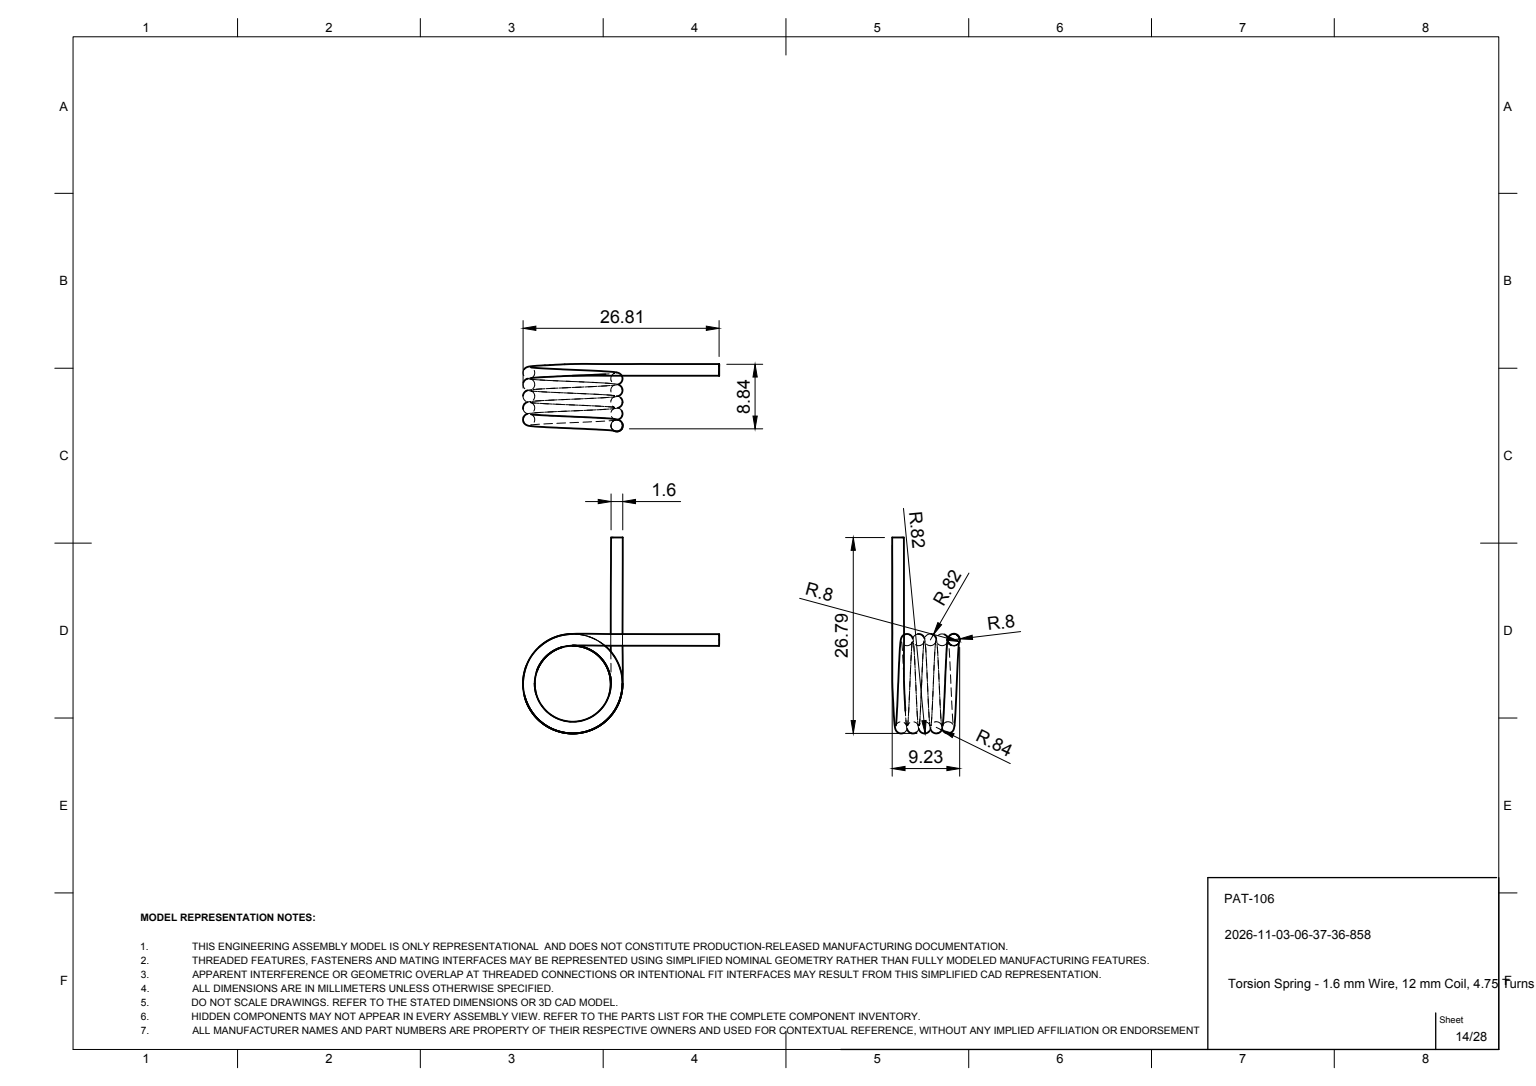
ISO-10303-21;
HEADER;
/* Generated by software containing ST-Developer
 * from STEP Tools, Inc. (www.steptools.com) 
 */

FILE_DESCRIPTION(
/* description */ ('Torsion-spring ratchet demonstrator'),
/* implementation_level */ '2;1');

FILE_NAME(
/* name */ 'Torsion Spring - 1.6 mm Wire, 12 mm Coil, 4.75 Turns.step',
/* time_stamp */ '2026-10-29T17:29:17-07:00',
/* author */ (''),
/* organization */ (''),
/* preprocessor_version */ 'ST-DEVELOPER v20.2',
/* originating_system */ 'Autodesk Translation Framework v15.17.0.0',
/* authorisation */ '');

FILE_SCHEMA (('AUTOMOTIVE_DESIGN { 1 0 10303 214 3 1 1 }'));
ENDSEC;

DATA;
#10=MECHANICAL_DESIGN_GEOMETRIC_PRESENTATION_REPRESENTATION('',(#307),#11258);
#11=B_SPLINE_SURFACE_WITH_KNOTS('',3,3,((#8927,#8928,#8929,#8930,#8931,
#8932,#8933,#8934,#8935,#8936,#8937,#8938,#8939,#8940,#8941,#8942,#8943,
#8944,#8945,#8946,#8947,#8948,#8949,#8950,#8951,#8952,#8953,#8954,#8955,
#8956,#8957,#8958,#8959,#8960,#8961,#8962,#8963,#8964,#8965,#8966,#8967,
#8968,#8969,#8970,#8971,#8972,#8973,#8974,#8975,#8976,#8977,#8978,#8979,
#8980,#8981,#8982,#8983,#8984,#8985,#8986,#8987,#8988,#8989,#8990,#8991,
#8992,#8993),(#8994,#8995,#8996,#8997,#8998,#8999,#9000,#9001,#9002,#9003,
#9004,#9005,#9006,#9007,#9008,#9009,#9010,#9011,#9012,#9013,#9014,#9015,
#9016,#9017,#9018,#9019,#9020,#9021,#9022,#9023,#9024,#9025,#9026,#9027,
#9028,#9029,#9030,#9031,#9032,#9033,#9034,#9035,#9036,#9037,#9038,#9039,
#9040,#9041,#9042,#9043,#9044,#9045,#9046,#9047,#9048,#9049,#9050,#9051,
#9052,#9053,#9054,#9055,#9056,#9057,#9058,#9059,#9060),(#9061,#9062,#9063,
#9064,#9065,#9066,#9067,#9068,#9069,#9070,#9071,#9072,#9073,#9074,#9075,
#9076,#9077,#9078,#9079,#9080,#9081,#9082,#9083,#9084,#9085,#9086,#9087,
#9088,#9089,#9090,#9091,#9092,#9093,#9094,#9095,#9096,#9097,#9098,#9099,
#9100,#9101,#9102,#9103,#9104,#9105,#9106,#9107,#9108,#9109,#9110,#9111,
#9112,#9113,#9114,#9115,#9116,#9117,#9118,#9119,#9120,#9121,#9122,#9123,
#9124,#9125,#9126,#9127),(#9128,#9129,#9130,#9131,#9132,#9133,#9134,#9135,
#9136,#9137,#9138,#9139,#9140,#9141,#9142,#9143,#9144,#9145,#9146,#9147,
#9148,#9149,#9150,#9151,#9152,#9153,#9154,#9155,#9156,#9157,#9158,#9159,
#9160,#9161,#9162,#9163,#9164,#9165,#9166,#9167,#9168,#9169,#9170,#9171,
#9172,#9173,#9174,#9175,#9176,#9177,#9178,#9179,#9180,#9181,#9182,#9183,
#9184,#9185,#9186,#9187,#9188,#9189,#9190,#9191,#9192,#9193,#9194),(#9195,
#9196,#9197,#9198,#9199,#9200,#9201,#9202,#9203,#9204,#9205,#9206,#9207,
#9208,#9209,#9210,#9211,#9212,#9213,#9214,#9215,#9216,#9217,#9218,#9219,
#9220,#9221,#9222,#9223,#9224,#9225,#9226,#9227,#9228,#9229,#9230,#9231,
#9232,#9233,#9234,#9235,#9236,#9237,#9238,#9239,#9240,#9241,#9242,#9243,
#9244,#9245,#9246,#9247,#9248,#9249,#9250,#9251,#9252,#9253,#9254,#9255,
#9256,#9257,#9258,#9259,#9260,#9261),(#9262,#9263,#9264,#9265,#9266,#9267,
#9268,#9269,#9270,#9271,#9272,#9273,#9274,#9275,#9276,#9277,#9278,#9279,
#9280,#9281,#9282,#9283,#9284,#9285,#9286,#9287,#9288,#9289,#9290,#9291,
#9292,#9293,#9294,#9295,#9296,#9297,#9298,#9299,#9300,#9301,#9302,#9303,
#9304,#9305,#9306,#9307,#9308,#9309,#9310,#9311,#9312,#9313,#9314,#9315,
#9316,#9317,#9318,#9319,#9320,#9321,#9322,#9323,#9324,#9325,#9326,#9327,
#9328),(#9329,#9330,#9331,#9332,#9333,#9334,#9335,#9336,#9337,#9338,#9339,
#9340,#9341,#9342,#9343,#9344,#9345,#9346,#9347,#9348,#9349,#9350,#9351,
#9352,#9353,#9354,#9355,#9356,#9357,#9358,#9359,#9360,#9361,#9362,#9363,
#9364,#9365,#9366,#9367,#9368,#9369,#9370,#9371,#9372,#9373,#9374,#9375,
#9376,#9377,#9378,#9379,#9380,#9381,#9382,#9383,#9384,#9385,#9386,#9387,
#9388,#9389,#9390,#9391,#9392,#9393,#9394,#9395),(#9396,#9397,#9398,#9399,
#9400,#9401,#9402,#9403,#9404,#9405,#9406,#9407,#9408,#9409,#9410,#9411,
#9412,#9413,#9414,#9415,#9416,#9417,#9418,#9419,#9420,#9421,#9422,#9423,
#9424,#9425,#9426,#9427,#9428,#9429,#9430,#9431,#9432,#9433,#9434,#9435,
#9436,#9437,#9438,#9439,#9440,#9441,#9442,#9443,#9444,#9445,#9446,#9447,
#9448,#9449,#9450,#9451,#9452,#9453,#9454,#9455,#9456,#9457,#9458,#9459,
#9460,#9461,#9462),(#9463,#9464,#9465,#9466,#9467,#9468,#9469,#9470,#9471,
#9472,#9473,#9474,#9475,#9476,#9477,#9478,#9479,#9480,#9481,#9482,#9483,
#9484,#9485,#9486,#9487,#9488,#9489,#9490,#9491,#9492,#9493,#9494,#9495,
#9496,#9497,#9498,#9499,#9500,#9501,#9502,#9503,#9504,#9505,#9506,#9507,
#9508,#9509,#9510,#9511,#9512,#9513,#9514,#9515,#9516,#9517,#9518,#9519,
#9520,#9521,#9522,#9523,#9524,#9525,#9526,#9527,#9528,#9529)),
 .UNSPECIFIED.,.F.,.F.,.F.,(4,1,1,1,1,1,4),(4,1,1,1,1,1,1,1,1,1,1,1,1,1,
1,1,1,1,1,1,1,1,1,1,1,1,1,1,1,1,1,1,1,1,1,1,1,1,1,1,1,1,1,1,1,1,1,1,1,1,
1,1,1,1,1,1,1,1,1,1,1,1,1,1,4),(-2.2472005777546,-1.52802098913967,-0.808841400524738,
-0.329388341448117,0.150064717628504,0.629517776705124,1.10897083578174),
(0.,0.0178571428571429,0.0357142857142857,0.0446428571428571,0.0535714285714286,
0.0625,0.0714285714285714,0.0803571428571428,0.0848214285714286,0.0892857142857143,
0.0982142857142857,0.107142857142857,0.125,0.142857142857143,0.166666666666667,
0.19047619047619,0.214285714285714,0.232142857142857,0.25,0.267857142857143,
0.285714285714286,0.303571428571429,0.321428571428571,0.339285714285714,
0.357142857142857,0.369047619047619,0.392857142857143,0.410714285714286,
0.428571428571429,0.452380952380952,0.476190476190476,0.492063492063492,
0.507936507936508,0.523809523809524,0.547619047619048,0.571428571428571,
0.595238095238095,0.619047619047619,0.642857142857143,0.666666666666667,
0.682539682539682,0.698412698412698,0.714285714285714,0.73015873015873,
0.746031746031746,0.761904761904762,0.785714285714286,0.809523809523809,
0.833333333333333,0.857142857142857,0.861607142857143,0.866071428571429,
0.875,0.892857142857143,0.901785714285714,0.910714285714286,0.915178571428571,
0.919642857142857,0.928571428571429,0.9375,0.946428571428571,0.955357142857143,
0.964285714285714,0.982142857142857,1.),.UNSPECIFIED.);
#12=B_SPLINE_SURFACE_WITH_KNOTS('',3,3,((#9670,#9671,#9672,#9673,#9674,
#9675,#9676,#9677,#9678,#9679,#9680,#9681,#9682,#9683,#9684,#9685,#9686,
#9687,#9688,#9689,#9690,#9691,#9692,#9693,#9694,#9695,#9696,#9697,#9698,
#9699,#9700,#9701,#9702,#9703,#9704,#9705,#9706,#9707,#9708,#9709,#9710,
#9711,#9712,#9713,#9714,#9715,#9716,#9717,#9718,#9719,#9720,#9721,#9722,
#9723,#9724,#9725,#9726,#9727,#9728,#9729,#9730,#9731,#9732,#9733,#9734,
#9735,#9736,#9737,#9738,#9739,#9740),(#9741,#9742,#9743,#9744,#9745,#9746,
#9747,#9748,#9749,#9750,#9751,#9752,#9753,#9754,#9755,#9756,#9757,#9758,
#9759,#9760,#9761,#9762,#9763,#9764,#9765,#9766,#9767,#9768,#9769,#9770,
#9771,#9772,#9773,#9774,#9775,#9776,#9777,#9778,#9779,#9780,#9781,#9782,
#9783,#9784,#9785,#9786,#9787,#9788,#9789,#9790,#9791,#9792,#9793,#9794,
#9795,#9796,#9797,#9798,#9799,#9800,#9801,#9802,#9803,#9804,#9805,#9806,
#9807,#9808,#9809,#9810,#9811),(#9812,#9813,#9814,#9815,#9816,#9817,#9818,
#9819,#9820,#9821,#9822,#9823,#9824,#9825,#9826,#9827,#9828,#9829,#9830,
#9831,#9832,#9833,#9834,#9835,#9836,#9837,#9838,#9839,#9840,#9841,#9842,
#9843,#9844,#9845,#9846,#9847,#9848,#9849,#9850,#9851,#9852,#9853,#9854,
#9855,#9856,#9857,#9858,#9859,#9860,#9861,#9862,#9863,#9864,#9865,#9866,
#9867,#9868,#9869,#9870,#9871,#9872,#9873,#9874,#9875,#9876,#9877,#9878,
#9879,#9880,#9881,#9882),(#9883,#9884,#9885,#9886,#9887,#9888,#9889,#9890,
#9891,#9892,#9893,#9894,#9895,#9896,#9897,#9898,#9899,#9900,#9901,#9902,
#9903,#9904,#9905,#9906,#9907,#9908,#9909,#9910,#9911,#9912,#9913,#9914,
#9915,#9916,#9917,#9918,#9919,#9920,#9921,#9922,#9923,#9924,#9925,#9926,
#9927,#9928,#9929,#9930,#9931,#9932,#9933,#9934,#9935,#9936,#9937,#9938,
#9939,#9940,#9941,#9942,#9943,#9944,#9945,#9946,#9947,#9948,#9949,#9950,
#9951,#9952,#9953)),.UNSPECIFIED.,.F.,.F.,.F.,(4,4),(4,1,1,1,1,1,1,1,1,
1,1,1,1,1,1,1,1,1,1,1,1,1,1,1,1,1,1,1,1,1,1,1,1,1,1,1,1,1,1,1,1,1,1,1,1,
1,1,1,1,1,1,1,1,1,1,1,1,1,1,1,1,1,1,1,1,1,1,1,4),(3.14159265358979,4.03598472942499),
(0.,0.0178571428571429,0.0357142857142857,0.0446428571428571,0.0535714285714286,
0.0625,0.0714285714285714,0.0803571428571428,0.0892857142857143,0.0982142857142857,
0.107142857142857,0.125,0.142857142857143,0.166666666666667,0.19047619047619,
0.196428571428571,0.214285714285714,0.232142857142857,0.25,0.267857142857143,
0.285714285714286,0.303571428571429,0.321428571428571,0.339285714285714,
0.357142857142857,0.369047619047619,0.392857142857143,0.410714285714286,
0.419642857142857,0.428571428571429,0.452380952380952,0.476190476190476,
0.492063492063492,0.5,0.507936507936508,0.523809523809524,0.547619047619048,
0.571428571428571,0.595238095238095,0.619047619047619,0.642857142857143,
0.666666666666667,0.682539682539682,0.698412698412698,0.714285714285714,
0.722222222222222,0.73015873015873,0.746031746031746,0.761904761904762,
0.773809523809524,0.785714285714286,0.809523809523809,0.833333333333333,
0.857142857142857,0.859375,0.861607142857143,0.866071428571429,0.875,0.892857142857143,
0.901785714285714,0.910714285714286,0.919642857142857,0.928571428571429,
0.9375,0.946428571428571,0.955357142857143,0.964285714285714,0.982142857142857,
1.),.UNSPECIFIED.);
#13=B_SPLINE_SURFACE_WITH_KNOTS('',3,3,((#10029,#10030,#10031,#10032,#10033,
#10034,#10035,#10036,#10037,#10038,#10039,#10040,#10041,#10042,#10043,#10044,
#10045,#10046,#10047,#10048,#10049,#10050,#10051,#10052,#10053,#10054,#10055,
#10056,#10057,#10058,#10059,#10060,#10061,#10062,#10063,#10064,#10065,#10066,
#10067,#10068,#10069,#10070,#10071,#10072,#10073,#10074,#10075,#10076,#10077,
#10078,#10079,#10080,#10081,#10082,#10083,#10084,#10085,#10086,#10087,#10088,
#10089,#10090,#10091,#10092,#10093,#10094,#10095,#10096,#10097,#10098,#10099,
#10100),(#10101,#10102,#10103,#10104,#10105,#10106,#10107,#10108,#10109,
#10110,#10111,#10112,#10113,#10114,#10115,#10116,#10117,#10118,#10119,#10120,
#10121,#10122,#10123,#10124,#10125,#10126,#10127,#10128,#10129,#10130,#10131,
#10132,#10133,#10134,#10135,#10136,#10137,#10138,#10139,#10140,#10141,#10142,
#10143,#10144,#10145,#10146,#10147,#10148,#10149,#10150,#10151,#10152,#10153,
#10154,#10155,#10156,#10157,#10158,#10159,#10160,#10161,#10162,#10163,#10164,
#10165,#10166,#10167,#10168,#10169,#10170,#10171,#10172),(#10173,#10174,
#10175,#10176,#10177,#10178,#10179,#10180,#10181,#10182,#10183,#10184,#10185,
#10186,#10187,#10188,#10189,#10190,#10191,#10192,#10193,#10194,#10195,#10196,
#10197,#10198,#10199,#10200,#10201,#10202,#10203,#10204,#10205,#10206,#10207,
#10208,#10209,#10210,#10211,#10212,#10213,#10214,#10215,#10216,#10217,#10218,
#10219,#10220,#10221,#10222,#10223,#10224,#10225,#10226,#10227,#10228,#10229,
#10230,#10231,#10232,#10233,#10234,#10235,#10236,#10237,#10238,#10239,#10240,
#10241,#10242,#10243,#10244),(#10245,#10246,#10247,#10248,#10249,#10250,
#10251,#10252,#10253,#10254,#10255,#10256,#10257,#10258,#10259,#10260,#10261,
#10262,#10263,#10264,#10265,#10266,#10267,#10268,#10269,#10270,#10271,#10272,
#10273,#10274,#10275,#10276,#10277,#10278,#10279,#10280,#10281,#10282,#10283,
#10284,#10285,#10286,#10287,#10288,#10289,#10290,#10291,#10292,#10293,#10294,
#10295,#10296,#10297,#10298,#10299,#10300,#10301,#10302,#10303,#10304,#10305,
#10306,#10307,#10308,#10309,#10310,#10311,#10312,#10313,#10314,#10315,#10316),
(#10317,#10318,#10319,#10320,#10321,#10322,#10323,#10324,#10325,#10326,
#10327,#10328,#10329,#10330,#10331,#10332,#10333,#10334,#10335,#10336,#10337,
#10338,#10339,#10340,#10341,#10342,#10343,#10344,#10345,#10346,#10347,#10348,
#10349,#10350,#10351,#10352,#10353,#10354,#10355,#10356,#10357,#10358,#10359,
#10360,#10361,#10362,#10363,#10364,#10365,#10366,#10367,#10368,#10369,#10370,
#10371,#10372,#10373,#10374,#10375,#10376,#10377,#10378,#10379,#10380,#10381,
#10382,#10383,#10384,#10385,#10386,#10387,#10388),(#10389,#10390,#10391,
#10392,#10393,#10394,#10395,#10396,#10397,#10398,#10399,#10400,#10401,#10402,
#10403,#10404,#10405,#10406,#10407,#10408,#10409,#10410,#10411,#10412,#10413,
#10414,#10415,#10416,#10417,#10418,#10419,#10420,#10421,#10422,#10423,#10424,
#10425,#10426,#10427,#10428,#10429,#10430,#10431,#10432,#10433,#10434,#10435,
#10436,#10437,#10438,#10439,#10440,#10441,#10442,#10443,#10444,#10445,#10446,
#10447,#10448,#10449,#10450,#10451,#10452,#10453,#10454,#10455,#10456,#10457,
#10458,#10459,#10460)),.UNSPECIFIED.,.F.,.F.,.F.,(4,1,1,4),(4,1,1,1,1,1,
1,1,1,1,1,1,1,1,1,1,1,1,1,1,1,1,1,1,1,1,1,1,1,1,1,1,1,1,1,1,1,1,1,1,1,1,
1,1,1,1,1,1,1,1,1,1,1,1,1,1,1,1,1,1,1,1,1,1,1,1,1,1,1,4),(1.10897083578174,
1.98009447198525,2.56084356278759,3.14159265358993),(0.,0.0178571428571429,
0.0357142857142857,0.0446428571428571,0.0535714285714286,0.0625,0.0714285714285714,
0.0803571428571428,0.0848214285714286,0.0892857142857143,0.0982142857142857,
0.107142857142857,0.125,0.142857142857143,0.166666666666667,0.19047619047619,
0.196428571428571,0.214285714285714,0.232142857142857,0.25,0.267857142857143,
0.285714285714286,0.303571428571429,0.321428571428571,0.339285714285714,
0.357142857142857,0.369047619047619,0.392857142857143,0.410714285714286,
0.419642857142857,0.428571428571429,0.452380952380952,0.476190476190476,
0.492063492063492,0.507936507936508,0.523809523809524,0.547619047619048,
0.571428571428571,0.595238095238095,0.619047619047619,0.642857142857143,
0.666666666666667,0.682539682539682,0.698412698412698,0.714285714285714,
0.73015873015873,0.746031746031746,0.761904761904762,0.773809523809524,
0.785714285714286,0.791666666666667,0.809523809523809,0.833333333333333,
0.857142857142857,0.859375,0.861607142857143,0.866071428571429,0.875,0.892857142857143,
0.901785714285714,0.910714285714286,0.915178571428571,0.919642857142857,
0.928571428571429,0.9375,0.946428571428571,0.955357142857143,0.964285714285714,
0.982142857142857,1.),.UNSPECIFIED.);
#223=B_SPLINE_CURVE_WITH_KNOTS('',3,(#9532,#9533,#9534,#9535,#9536,#9537,
#9538,#9539,#9540,#9541,#9542,#9543,#9544,#9545,#9546,#9547,#9548,#9549,
#9550,#9551,#9552,#9553,#9554,#9555,#9556,#9557,#9558,#9559,#9560,#9561,
#9562,#9563,#9564,#9565,#9566,#9567,#9568,#9569,#9570,#9571,#9572,#9573,
#9574,#9575,#9576,#9577,#9578,#9579,#9580,#9581,#9582,#9583,#9584,#9585,
#9586,#9587,#9588,#9589,#9590,#9591,#9592,#9593,#9594,#9595,#9596,#9597,
#9598),.UNSPECIFIED.,.F.,.F.,(4,1,1,1,1,1,1,1,1,1,1,1,1,1,1,1,1,1,1,1,1,
1,1,1,1,1,1,1,1,1,1,1,1,1,1,1,1,1,1,1,1,1,1,1,1,1,1,1,1,1,1,1,1,1,1,1,1,
1,1,1,1,1,1,1,4),(-1.,-0.982142857142857,-0.964285714285714,-0.955357142857143,
-0.946428571428571,-0.9375,-0.928571428571429,-0.919642857142857,-0.915178571428571,
-0.910714285714286,-0.901785714285714,-0.892857142857143,-0.875,-0.866071428571429,
-0.861607142857143,-0.857142857142857,-0.833333333333333,-0.809523809523809,
-0.785714285714286,-0.761904761904762,-0.746031746031746,-0.73015873015873,
-0.714285714285714,-0.698412698412698,-0.682539682539682,-0.666666666666667,
-0.642857142857143,-0.619047619047619,-0.595238095238095,-0.571428571428571,
-0.547619047619048,-0.523809523809524,-0.507936507936508,-0.492063492063492,
-0.476190476190476,-0.452380952380952,-0.428571428571429,-0.410714285714286,
-0.392857142857143,-0.369047619047619,-0.357142857142857,-0.339285714285714,
-0.321428571428571,-0.303571428571429,-0.285714285714286,-0.267857142857143,
-0.25,-0.232142857142857,-0.214285714285714,-0.19047619047619,-0.166666666666667,
-0.142857142857143,-0.125,-0.107142857142857,-0.0982142857142857,-0.0892857142857143,
-0.0848214285714286,-0.0803571428571428,-0.0714285714285714,-0.0625,-0.0535714285714286,
-0.0446428571428571,-0.0357142857142857,-0.0178571428571429,0.),
 .UNSPECIFIED.);
#224=B_SPLINE_CURVE_WITH_KNOTS('',3,(#9602,#9603,#9604,#9605,#9606,#9607,
#9608,#9609,#9610,#9611,#9612,#9613,#9614,#9615,#9616,#9617,#9618,#9619,
#9620,#9621,#9622,#9623,#9624,#9625,#9626,#9627,#9628,#9629,#9630,#9631,
#9632,#9633,#9634,#9635,#9636,#9637,#9638,#9639,#9640,#9641,#9642,#9643,
#9644,#9645,#9646,#9647,#9648,#9649,#9650,#9651,#9652,#9653,#9654,#9655,
#9656,#9657,#9658,#9659,#9660,#9661,#9662,#9663,#9664,#9665,#9666,#9667,
#9668),.UNSPECIFIED.,.F.,.F.,(4,1,1,1,1,1,1,1,1,1,1,1,1,1,1,1,1,1,1,1,1,
1,1,1,1,1,1,1,1,1,1,1,1,1,1,1,1,1,1,1,1,1,1,1,1,1,1,1,1,1,1,1,1,1,1,1,1,
1,1,1,1,1,1,1,4),(-1.,-0.982142857142857,-0.964285714285714,-0.955357142857143,
-0.946428571428571,-0.9375,-0.928571428571429,-0.919642857142857,-0.915178571428571,
-0.910714285714286,-0.901785714285714,-0.892857142857143,-0.875,-0.866071428571429,
-0.861607142857143,-0.857142857142857,-0.833333333333333,-0.809523809523809,
-0.785714285714286,-0.761904761904762,-0.746031746031746,-0.73015873015873,
-0.714285714285714,-0.698412698412698,-0.682539682539682,-0.666666666666667,
-0.642857142857143,-0.619047619047619,-0.595238095238095,-0.571428571428571,
-0.547619047619048,-0.523809523809524,-0.507936507936508,-0.492063492063492,
-0.476190476190476,-0.452380952380952,-0.428571428571429,-0.410714285714286,
-0.392857142857143,-0.369047619047619,-0.357142857142857,-0.339285714285714,
-0.321428571428571,-0.303571428571429,-0.285714285714286,-0.267857142857143,
-0.25,-0.232142857142857,-0.214285714285714,-0.19047619047619,-0.166666666666667,
-0.142857142857143,-0.125,-0.107142857142857,-0.0982142857142857,-0.0892857142857143,
-0.0848214285714286,-0.0803571428571428,-0.0714285714285714,-0.0625,-0.0535714285714286,
-0.0446428571428571,-0.0357142857142857,-0.0178571428571429,0.),
 .UNSPECIFIED.);
#225=B_SPLINE_CURVE_WITH_KNOTS('',3,(#9957,#9958,#9959,#9960,#9961,#9962,
#9963,#9964,#9965,#9966,#9967,#9968,#9969,#9970,#9971,#9972,#9973,#9974,
#9975,#9976,#9977,#9978,#9979,#9980,#9981,#9982,#9983,#9984,#9985,#9986,
#9987,#9988,#9989,#9990,#9991,#9992,#9993,#9994,#9995,#9996,#9997,#9998,
#9999,#10000,#10001,#10002,#10003,#10004,#10005,#10006,#10007,#10008,#10009,
#10010,#10011,#10012,#10013,#10014,#10015,#10016,#10017,#10018,#10019,#10020,
#10021,#10022,#10023,#10024,#10025,#10026,#10027),.UNSPECIFIED.,.F.,.F.,
(4,1,1,1,1,1,1,1,1,1,1,1,1,1,1,1,1,1,1,1,1,1,1,1,1,1,1,1,1,1,1,1,1,1,1,
1,1,1,1,1,1,1,1,1,1,1,1,1,1,1,1,1,1,1,1,1,1,1,1,1,1,1,1,1,1,1,1,1,4),(0.,
0.0178571428571429,0.0357142857142857,0.0446428571428571,0.0535714285714286,
0.0625,0.0714285714285714,0.0803571428571428,0.0892857142857143,0.0982142857142857,
0.107142857142857,0.125,0.142857142857143,0.166666666666667,0.19047619047619,
0.196428571428571,0.214285714285714,0.232142857142857,0.25,0.267857142857143,
0.285714285714286,0.303571428571429,0.321428571428571,0.339285714285714,
0.357142857142857,0.369047619047619,0.392857142857143,0.410714285714286,
0.419642857142857,0.428571428571429,0.452380952380952,0.476190476190476,
0.492063492063492,0.5,0.507936507936508,0.523809523809524,0.547619047619048,
0.571428571428571,0.595238095238095,0.619047619047619,0.642857142857143,
0.666666666666667,0.682539682539682,0.698412698412698,0.714285714285714,
0.722222222222222,0.73015873015873,0.746031746031746,0.761904761904762,
0.773809523809524,0.785714285714286,0.809523809523809,0.833333333333333,
0.857142857142857,0.859375,0.861607142857143,0.866071428571429,0.875,0.892857142857143,
0.901785714285714,0.910714285714286,0.919642857142857,0.928571428571429,
0.9375,0.946428571428571,0.955357142857143,0.964285714285714,0.982142857142857,
1.),.UNSPECIFIED.);
#251=SHAPE_REPRESENTATION_RELATIONSHIP('SRR','None',#11378,#275);
#275=ADVANCED_BREP_SHAPE_REPRESENTATION('',(#337),#11248);
#307=STYLED_ITEM('',(#11584),#337);
#337=MANIFOLD_SOLID_BREP('Body1',#5180);
#528=PLANE('',#5869);
#529=PLANE('',#5870);
#810=FACE_OUTER_BOUND('',#1190,.T.);
#811=FACE_OUTER_BOUND('',#1191,.T.);
#812=FACE_OUTER_BOUND('',#1192,.T.);
#813=FACE_OUTER_BOUND('',#1193,.T.);
#814=FACE_OUTER_BOUND('',#1194,.T.);
#1190=EDGE_LOOP('',(#4194,#4195,#4196,#4197));
#1191=EDGE_LOOP('',(#4198,#4199,#4200,#4201));
#1192=EDGE_LOOP('',(#4202,#4203,#4204,#4205));
#1193=EDGE_LOOP('',(#4206,#4207,#4208));
#1194=EDGE_LOOP('',(#4209,#4210,#4211));
#2289=CIRCLE('',#5863,0.08);
#2290=CIRCLE('',#5864,0.08);
#2291=CIRCLE('',#5865,0.08);
#2292=CIRCLE('',#5866,0.08);
#2293=CIRCLE('',#5867,0.08);
#2294=CIRCLE('',#5868,0.08);
#2593=VERTEX_POINT('',#9530);
#2594=VERTEX_POINT('',#9531);
#2595=VERTEX_POINT('',#9599);
#2596=VERTEX_POINT('',#9601);
#2597=VERTEX_POINT('',#9954);
#2598=VERTEX_POINT('',#9956);
#3157=EDGE_CURVE('',#2593,#2594,#223,.T.);
#3158=EDGE_CURVE('',#2595,#2593,#2289,.T.);
#3159=EDGE_CURVE('',#2595,#2596,#224,.T.);
#3160=EDGE_CURVE('',#2596,#2594,#2290,.T.);
#3161=EDGE_CURVE('',#2597,#2595,#2291,.T.);
#3162=EDGE_CURVE('',#2598,#2597,#225,.T.);
#3163=EDGE_CURVE('',#2598,#2596,#2292,.T.);
#3164=EDGE_CURVE('',#2594,#2598,#2293,.T.);
#3165=EDGE_CURVE('',#2593,#2597,#2294,.T.);
#4194=ORIENTED_EDGE('',*,*,#3157,.F.);
#4195=ORIENTED_EDGE('',*,*,#3158,.F.);
#4196=ORIENTED_EDGE('',*,*,#3159,.T.);
#4197=ORIENTED_EDGE('',*,*,#3160,.T.);
#4198=ORIENTED_EDGE('',*,*,#3159,.F.);
#4199=ORIENTED_EDGE('',*,*,#3161,.F.);
#4200=ORIENTED_EDGE('',*,*,#3162,.F.);
#4201=ORIENTED_EDGE('',*,*,#3163,.T.);
#4202=ORIENTED_EDGE('',*,*,#3157,.T.);
#4203=ORIENTED_EDGE('',*,*,#3164,.T.);
#4204=ORIENTED_EDGE('',*,*,#3162,.T.);
#4205=ORIENTED_EDGE('',*,*,#3165,.F.);
#4206=ORIENTED_EDGE('',*,*,#3161,.T.);
#4207=ORIENTED_EDGE('',*,*,#3158,.T.);
#4208=ORIENTED_EDGE('',*,*,#3165,.T.);
#4209=ORIENTED_EDGE('',*,*,#3163,.F.);
#4210=ORIENTED_EDGE('',*,*,#3164,.F.);
#4211=ORIENTED_EDGE('',*,*,#3160,.F.);
#5036=ADVANCED_FACE('',(#810),#11,.T.);
#5037=ADVANCED_FACE('',(#811),#12,.T.);
#5038=ADVANCED_FACE('',(#812),#13,.T.);
#5039=ADVANCED_FACE('',(#813),#528,.T.);
#5040=ADVANCED_FACE('',(#814),#529,.F.);
#5180=CLOSED_SHELL('',(#5036,#5037,#5038,#5039,#5040));
#5862=AXIS2_PLACEMENT_3D('',#8926,#7040,#7041);
#5863=AXIS2_PLACEMENT_3D('',#9600,#7042,#7043);
#5864=AXIS2_PLACEMENT_3D('',#9669,#7044,#7045);
#5865=AXIS2_PLACEMENT_3D('',#9955,#7046,#7047);
#5866=AXIS2_PLACEMENT_3D('',#10028,#7048,#7049);
#5867=AXIS2_PLACEMENT_3D('',#10461,#7050,#7051);
#5868=AXIS2_PLACEMENT_3D('',#10462,#7052,#7053);
#5869=AXIS2_PLACEMENT_3D('',#10463,#7054,#7055);
#5870=AXIS2_PLACEMENT_3D('',#10464,#7056,#7057);
#7040=DIRECTION('axis',(0.,0.,1.));
#7041=DIRECTION('refdir',(1.,0.,0.));
#7042=DIRECTION('center_axis',(0.999998225160355,-0.00106218492982768,0.00155609746344814));
#7043=DIRECTION('ref_axis',(-0.00116547091797426,0.300191357997798,0.953878289018561));
#7044=DIRECTION('center_axis',(0.00155609740738298,-0.0010621849112801,
0.999998225160462));
#7045=DIRECTION('ref_axis',(-0.00155444353908754,0.999998225160461,0.0010646037811343));
#7046=DIRECTION('center_axis',(0.999998225160355,-0.00106218492982768,0.00155609746344814));
#7047=DIRECTION('ref_axis',(-0.00116547091797426,0.300191357997798,0.953878289018561));
#7048=DIRECTION('center_axis',(0.00155609740738298,-0.0010621849112801,
0.999998225160462));
#7049=DIRECTION('ref_axis',(-0.00155444353908754,0.999998225160461,0.0010646037811343));
#7050=DIRECTION('center_axis',(0.00155609740738298,-0.0010621849112801,
0.999998225160462));
#7051=DIRECTION('ref_axis',(-0.00155444353908754,0.999998225160461,0.0010646037811343));
#7052=DIRECTION('center_axis',(0.999998225160355,-0.00106218492982768,0.00155609746344814));
#7053=DIRECTION('ref_axis',(-0.00116547091797426,0.300191357997798,0.953878289018561));
#7054=DIRECTION('center_axis',(0.999998225160355,-0.00106218492982768,0.00155609746344814));
#7055=DIRECTION('ref_axis',(-0.00116547091797426,0.300191357997798,0.953878289018561));
#7056=DIRECTION('center_axis',(0.00155609740738298,-0.0010621849112801,
0.999998225160462));
#7057=DIRECTION('ref_axis',(-0.00155444353908754,0.999998225160462,0.0010646037811343));
#8926=CARTESIAN_POINT('',(0.,0.,0.));
#8927=CARTESIAN_POINT('Ctrl Pts',(0.662463988280159,-0.0499822726657336,
-2.00015029073282));
#8928=CARTESIAN_POINT('Ctrl Pts',(0.662719098649113,-0.050156409826639,
-1.8362081654112));
#8929=CARTESIAN_POINT('Ctrl Pts',(0.661897332210143,-0.0496009500256405,
-1.51421284590545));
#8930=CARTESIAN_POINT('Ctrl Pts',(0.662849183916153,-0.050231417425612,
-1.10458538375921));
#8931=CARTESIAN_POINT('Ctrl Pts',(0.662676266642772,-0.050132523365314,
-0.778488486630415));
#8932=CARTESIAN_POINT('Ctrl Pts',(0.660820022877162,-0.0488315955858374,
-0.544415125004604));
#8933=CARTESIAN_POINT('Ctrl Pts',(0.663563470597623,-0.0508446374556383,
-0.288026483088336));
#8934=CARTESIAN_POINT('Ctrl Pts',(0.667640080240138,-0.0524139639419364,
-0.0320317672708526));
#8935=CARTESIAN_POINT('Ctrl Pts',(0.65335380658105,-0.0455068140358546,
0.139218056313768));
#8936=CARTESIAN_POINT('Ctrl Pts',(0.611163697009464,-0.0383525034286994,
0.264648815779984));
#8937=CARTESIAN_POINT('Ctrl Pts',(0.548065973192159,-0.032280894159065,
0.384307758714896));
#8938=CARTESIAN_POINT('Ctrl Pts',(0.431002395435098,-0.0256993836631372,
0.520971575878654));
#8939=CARTESIAN_POINT('Ctrl Pts',(0.191480329024041,-0.0134075415523006,
0.662765347245377));
#8940=CARTESIAN_POINT('Ctrl Pts',(-0.170310845287768,0.00096264921625724,
0.690490277729099));
#8941=CARTESIAN_POINT('Ctrl Pts',(-0.585085784735021,0.0207569079373872,
0.435755076168825));
#8942=CARTESIAN_POINT('Ctrl Pts',(-0.744693743478759,0.0422927786570434,
-0.0951523515529584));
#8943=CARTESIAN_POINT('Ctrl Pts',(-0.431538112822807,0.0659892634348224,
-0.617104732797172));
#8944=CARTESIAN_POINT('Ctrl Pts',(0.115758946274973,0.0876905285771165,
-0.725599039992233));
#8945=CARTESIAN_POINT('Ctrl Pts',(0.53747991286649,0.107478289621193,-0.475188997283933));
#8946=CARTESIAN_POINT('Ctrl Pts',(0.715006044039375,0.125301300434412,-0.0720347673296787));
#8947=CARTESIAN_POINT('Ctrl Pts',(0.622824528841228,0.143151007884386,0.360207879087552));
#8948=CARTESIAN_POINT('Ctrl Pts',(0.295215046776041,0.161020056779893,0.657018975821946));
#8949=CARTESIAN_POINT('Ctrl Pts',(-0.144725676703892,0.178909769816401,
0.70633098622582));
#8950=CARTESIAN_POINT('Ctrl Pts',(-0.530690929834931,0.196817259725453,
0.489300976461692));
#8951=CARTESIAN_POINT('Ctrl Pts',(-0.717478987054585,0.214742051156983,
0.086194632105411));
#8952=CARTESIAN_POINT('Ctrl Pts',(-0.641992299862074,0.230688881084643,
-0.299876917809462));
#8953=CARTESIAN_POINT('Ctrl Pts',(-0.36030002070441,0.248640851668397,-0.629569645495563));
#8954=CARTESIAN_POINT('Ctrl Pts',(0.0867941523773002,0.266605918529927,
-0.737064913155744));
#8955=CARTESIAN_POINT('Ctrl Pts',(0.522621279421028,0.286581789189134,-0.500819963452499));
#8956=CARTESIAN_POINT('Ctrl Pts',(0.740365136709862,0.306568406437996,-0.0577085025886233));
#8957=CARTESIAN_POINT('Ctrl Pts',(0.588086029972563,0.328565375698038,0.488053495238463));
#8958=CARTESIAN_POINT('Ctrl Pts',(0.0972167907293641,0.34990603829391,0.730574719890591));
#8959=CARTESIAN_POINT('Ctrl Pts',(-0.348606790473969,0.368583951861805,
0.625079898555237));
#8960=CARTESIAN_POINT('Ctrl Pts',(-0.625117601034868,0.384596133557627,
0.348183842295094));
#8961=CARTESIAN_POINT('Ctrl Pts',(-0.731235197502955,0.403278517609434,
-0.0977683708505558));
#8962=CARTESIAN_POINT('Ctrl Pts',(-0.487350453008389,0.424630334656425,
-0.588208599365547));
#8963=CARTESIAN_POINT('Ctrl Pts',(0.107586035230619,0.448648433132338,-0.756188390862319));
#8964=CARTESIAN_POINT('Ctrl Pts',(0.630965640778732,0.472660315479601,-0.429375166251397));
#8965=CARTESIAN_POINT('Ctrl Pts',(0.742175157663465,0.496662180030771,0.177201798791322));
#8966=CARTESIAN_POINT('Ctrl Pts',(0.367484330759339,0.520650735211898,0.667598289986901));
#8967=CARTESIAN_POINT('Ctrl Pts',(-0.1772094561828,0.541959207305282,0.714834645121414));
#8968=CARTESIAN_POINT('Ctrl Pts',(-0.55158365946692,0.56059094898577,0.452401551542145));
#8969=CARTESIAN_POINT('Ctrl Pts',(-0.707144881750632,0.57655098007586,0.0945309854926571));
#8970=CARTESIAN_POINT('Ctrl Pts',(-0.650080156703408,0.592499998475874,
-0.292288521076879));
#8971=CARTESIAN_POINT('Ctrl Pts',(-0.39813025511233,0.608437064253082,-0.590670145737896));
#8972=CARTESIAN_POINT('Ctrl Pts',(-0.0275908863199736,0.62436100859898,
-0.710669286038228));
#8973=CARTESIAN_POINT('Ctrl Pts',(0.414715655942592,0.642922729480766,-0.603621999120373));
#8974=CARTESIAN_POINT('Ctrl Pts',(0.73835387107679,0.664111160627632,-0.166965130048199));
#8975=CARTESIAN_POINT('Ctrl Pts',(0.620304111002753,0.687911568470837,0.433769461113443));
#8976=CARTESIAN_POINT('Ctrl Pts',(0.0958337440893244,0.711671376372341,
0.74830999711301));
#8977=CARTESIAN_POINT('Ctrl Pts',(-0.328971586153759,0.728968689390915,
0.621190836988033));
#8978=CARTESIAN_POINT('Ctrl Pts',(-0.510250580429896,0.739824441432273,
0.439145396424497));
#8979=CARTESIAN_POINT('Ctrl Pts',(-0.592478248153049,0.74570751472679,0.326342499792088));
#8980=CARTESIAN_POINT('Ctrl Pts',(-0.689058767063034,0.756222082569521,
0.0984146554749596));
#8981=CARTESIAN_POINT('Ctrl Pts',(-0.666219044663549,0.767653433960867,
-0.192704218915611));
#8982=CARTESIAN_POINT('Ctrl Pts',(-0.523816993927788,0.780063785948551,
-0.433645748061385));
#8983=CARTESIAN_POINT('Ctrl Pts',(-0.386340473147736,0.786669200591926,
-0.551372175845378));
#8984=CARTESIAN_POINT('Ctrl Pts',(-0.265956682682317,0.792781771671027,
-0.614881276898037));
#8985=CARTESIAN_POINT('Ctrl Pts',(-0.139596638836966,0.799988366367406,
-0.657366153595634));
#8986=CARTESIAN_POINT('Ctrl Pts',(0.0321180206196141,0.806907294366097,
-0.671653874643804));
#8987=CARTESIAN_POINT('Ctrl Pts',(0.288027302850487,0.805335668320584,-0.667586118918959));
#8988=CARTESIAN_POINT('Ctrl Pts',(0.54442707625171,0.8033242699894,-0.664844003722482));
#8989=CARTESIAN_POINT('Ctrl Pts',(0.778488091977107,0.804624888614752,-0.666703265676913));
#8990=CARTESIAN_POINT('Ctrl Pts',(1.10459263968738,0.804724235202262,-0.66687751216757));
#8991=CARTESIAN_POINT('Ctrl Pts',(1.51421119194035,0.804093904068503,-0.665928948647562));
#8992=CARTESIAN_POINT('Ctrl Pts',(1.83620821687538,0.804649660698633,-0.66675251787415));
#8993=CARTESIAN_POINT('Ctrl Pts',(2.00015071794412,0.804475523135573,-0.666497406911305));
#8994=CARTESIAN_POINT('Ctrl Pts',(0.674446082047605,-0.0350079680470159,
-2.0001530305623));
#8995=CARTESIAN_POINT('Ctrl Pts',(0.674701196382384,-0.0351821079149749,
-1.83620835667417));
#8996=CARTESIAN_POINT('Ctrl Pts',(0.673880936475708,-0.0346263233539259,
-1.51419872926041));
#8997=CARTESIAN_POINT('Ctrl Pts',(0.674833527244618,-0.0352575894449097,
-1.10460499764898));
#8998=CARTESIAN_POINT('Ctrl Pts',(0.674662892741623,-0.0351576445284815,
-0.778466545112985));
#8999=CARTESIAN_POINT('Ctrl Pts',(0.67280508837135,-0.0338589215885485,
-0.544434301215379));
#9000=CARTESIAN_POINT('Ctrl Pts',(0.675556714498639,-0.0358668037102216,
-0.288024615576321));
#9001=CARTESIAN_POINT('Ctrl Pts',(0.679620952141269,-0.0374476933188151,
-0.032249939480985));
#9002=CARTESIAN_POINT('Ctrl Pts',(0.665348834630966,-0.0305040167873278,
0.14048082279948));
#9003=CARTESIAN_POINT('Ctrl Pts',(0.62228669882739,-0.0231938376451895,
0.268666180783973));
#9004=CARTESIAN_POINT('Ctrl Pts',(0.557982182284105,-0.0170103722728659,
0.390533052942412));
#9005=CARTESIAN_POINT('Ctrl Pts',(0.438991286666523,-0.0103201349719665,
0.52946260531362));
#9006=CARTESIAN_POINT('Ctrl Pts',(0.195264943047363,0.00218717191725961,
0.673765355231291));
#9007=CARTESIAN_POINT('Ctrl Pts',(-0.172425934555583,0.0167901354760882,
0.701847369499063));
#9008=CARTESIAN_POINT('Ctrl Pts',(-0.593820028218252,0.0369011555335372,
0.443051917288691));
#9009=CARTESIAN_POINT('Ctrl Pts',(-0.755714874644402,0.0587598776212364,
-0.0959321206050264));
#9010=CARTESIAN_POINT('Ctrl Pts',(-0.43801433194566,0.0827940205198624,
-0.625251628852071));
#9011=CARTESIAN_POINT('Ctrl Pts',(0.116602046289419,0.104783098701226,-0.735092792907372));
#9012=CARTESIAN_POINT('Ctrl Pts',(0.543561315738589,0.124817673728603,-0.481501423919919));
#9013=CARTESIAN_POINT('Ctrl Pts',(0.723146404942936,0.142850573437901,-0.073564714561987));
#9014=CARTESIAN_POINT('Ctrl Pts',(0.629891273516298,0.160897879216403,0.363473014402678));
#9015=CARTESIAN_POINT('Ctrl Pts',(0.298840430266652,0.178952078689978,0.663337021281643));
#9016=CARTESIAN_POINT('Ctrl Pts',(-0.145370129699683,0.19701439207729,0.713079165107859));
#9017=CARTESIAN_POINT('Ctrl Pts',(-0.534777464258203,0.215081700570601,
0.494059450643713));
#9018=CARTESIAN_POINT('Ctrl Pts',(-0.723059497631479,0.233153598058585,
0.087604707943711));
#9019=CARTESIAN_POINT('Ctrl Pts',(-0.646967875903001,0.249219385062332,
-0.301358039243341));
#9020=CARTESIAN_POINT('Ctrl Pts',(-0.363297994601133,0.26729513369037,-0.633323883813959));
#9021=CARTESIAN_POINT('Ctrl Pts',(0.0865905388130023,0.285371192232844,
-0.741400774225685));
#9022=CARTESIAN_POINT('Ctrl Pts',(0.524706169760779,0.305452127192914,-0.503845943167671));
#9023=CARTESIAN_POINT('Ctrl Pts',(0.743402185160331,0.325530022126121,-0.058664817656703));
#9024=CARTESIAN_POINT('Ctrl Pts',(0.590448745665821,0.347606360017064,0.48909521564047));
#9025=CARTESIAN_POINT('Ctrl Pts',(0.0981851250008973,0.369004878005666,
0.732177168636611));
#9026=CARTESIAN_POINT('Ctrl Pts',(-0.348488468098564,0.387718276399827,
0.626441749101411));
#9027=CARTESIAN_POINT('Ctrl Pts',(-0.62532356257491,0.403750121631928,0.34916763101975));
#9028=CARTESIAN_POINT('Ctrl Pts',(-0.73146453597972,0.422443135444508,-0.0970695459087969));
#9029=CARTESIAN_POINT('Ctrl Pts',(-0.487535521710562,0.443787780507866,
-0.587339074779301));
#9030=CARTESIAN_POINT('Ctrl Pts',(0.106710568101606,0.467775062885446,-0.75498659819416));
#9031=CARTESIAN_POINT('Ctrl Pts',(0.628862026286412,0.49173208797649,-0.428789598129798));
#9032=CARTESIAN_POINT('Ctrl Pts',(0.739595803505217,0.515655142144853,0.175870704718188));
#9033=CARTESIAN_POINT('Ctrl Pts',(0.366376505463985,0.539541361351028,0.664120189316023));
#9034=CARTESIAN_POINT('Ctrl Pts',(-0.175506327148597,0.560738153809924,
0.711020492425908));
#9035=CARTESIAN_POINT('Ctrl Pts',(-0.54760485001816,0.579257515342459,0.450116428906716));
#9036=CARTESIAN_POINT('Ctrl Pts',(-0.702114990885751,0.595111390068342,
0.0946054547014213));
#9037=CARTESIAN_POINT('Ctrl Pts',(-0.645425496799589,0.610942449002933,
-0.289378750952378));
#9038=CARTESIAN_POINT('Ctrl Pts',(-0.395457432624221,0.626751558207065,
-0.585362642366029));
#9039=CARTESIAN_POINT('Ctrl Pts',(-0.0280797855644617,0.642538439860898,
-0.704297505820287));
#9040=CARTESIAN_POINT('Ctrl Pts',(0.410157779824956,0.660929008716659,-0.598194594147799));
#9041=CARTESIAN_POINT('Ctrl Pts',(0.730444289398745,0.681901601594788,-0.165864021920736));
#9042=CARTESIAN_POINT('Ctrl Pts',(0.613580247437332,0.705441153426337,0.428286178430747));
#9043=CARTESIAN_POINT('Ctrl Pts',(0.0952918314245258,0.72891509356906,0.738958605866823));
#9044=CARTESIAN_POINT('Ctrl Pts',(-0.324020729601473,0.745988444923654,
0.613400639649111));
#9045=CARTESIAN_POINT('Ctrl Pts',(-0.502873233709575,0.756698580939822,
0.433790954112853));
#9046=CARTESIAN_POINT('Ctrl Pts',(-0.583995235083359,0.762502876341029,
0.322496949785477));
#9047=CARTESIAN_POINT('Ctrl Pts',(-0.67925606222965,0.772870829077922,0.0977335101944516));
#9048=CARTESIAN_POINT('Ctrl Pts',(-0.65666377058204,0.784140125347959,-0.189261322798156));
#9049=CARTESIAN_POINT('Ctrl Pts',(-0.516444187283226,0.796361392235239,
-0.426530997573169));
#9050=CARTESIAN_POINT('Ctrl Pts',(-0.380942240338964,0.802871714443619,
-0.542569702523433));
#9051=CARTESIAN_POINT('Ctrl Pts',(-0.262525555833722,0.808884384740767,
-0.604997953335358));
#9052=CARTESIAN_POINT('Ctrl Pts',(-0.138595359825784,0.81595371167701,-0.646716670398854));
#9053=CARTESIAN_POINT('Ctrl Pts',(0.0319355517137274,0.822844653227088,
-0.661020222212807));
#9054=CARTESIAN_POINT('Ctrl Pts',(0.288093504695908,0.821281075632325,-0.656931006487794));
#9055=CARTESIAN_POINT('Ctrl Pts',(0.544427040001579,0.819265409799516,-0.654193021724466));
#9056=CARTESIAN_POINT('Ctrl Pts',(0.778506679323761,0.820567398055238,-0.65604695266566));
#9057=CARTESIAN_POINT('Ctrl Pts',(1.10459883628042,0.820665745979243,-0.656221018219063));
#9058=CARTESIAN_POINT('Ctrl Pts',(1.51421765241308,0.820035614746722,-0.6552683862334));
#9059=CARTESIAN_POINT('Ctrl Pts',(1.83620811434072,0.820590881682782,-0.656090536299704));
#9060=CARTESIAN_POINT('Ctrl Pts',(2.00015105938536,0.820416743648137,-0.655835424645988));
#9061=CARTESIAN_POINT('Ctrl Pts',(0.687145391337529,0.00388813180289089,
-2.00013147703594));
#9062=CARTESIAN_POINT('Ctrl Pts',(0.687400475859769,0.0037140122848332,
-1.83620596164366));
#9063=CARTESIAN_POINT('Ctrl Pts',(0.686580688274375,0.00426996159012147,
-1.51426120920445));
#9064=CARTESIAN_POINT('Ctrl Pts',(0.687528287675259,0.00363896296830716,
-1.10450912461653));
#9065=CARTESIAN_POINT('Ctrl Pts',(0.687361410679772,0.00373905286893215,
-0.778550764556369));
#9066=CARTESIAN_POINT('Ctrl Pts',(0.685492998268397,0.00503776682278646,
-0.544450526600379));
#9067=CARTESIAN_POINT('Ctrl Pts',(0.688265132824333,0.00303048983174741,
-0.287682055551203));
#9068=CARTESIAN_POINT('Ctrl Pts',(0.692275545237537,0.00144918010494716,
-0.0326506971997516));
#9069=CARTESIAN_POINT('Ctrl Pts',(0.67811721874054,0.00839277279208392,
0.140578602255062));
#9070=CARTESIAN_POINT('Ctrl Pts',(0.63417051039127,0.0158657021192725,0.271702248096095));
#9071=CARTESIAN_POINT('Ctrl Pts',(0.568467937345546,0.0221776380697667,
0.396075371092485));
#9072=CARTESIAN_POINT('Ctrl Pts',(0.447630344944513,0.0289704247052655,
0.537162845625327));
#9073=CARTESIAN_POINT('Ctrl Pts',(0.199876057358082,0.0416847890516129,
0.683850399068708));
#9074=CARTESIAN_POINT('Ctrl Pts',(-0.173340277410583,0.0565066590856592,
0.712241041234605));
#9075=CARTESIAN_POINT('Ctrl Pts',(-0.600363534440907,0.0768907360741932,
0.449858568469966));
#9076=CARTESIAN_POINT('Ctrl Pts',(-0.763917267702635,0.0990052380588372,
-0.0954913299225577));
#9077=CARTESIAN_POINT('Ctrl Pts',(-0.442946718272606,0.123269337596085,
-0.629705813071489));
#9078=CARTESIAN_POINT('Ctrl Pts',(0.115829754215989,0.14542261482116,-0.740117721914303));
#9079=CARTESIAN_POINT('Ctrl Pts',(0.545089263156225,0.16557013801192,-0.485003463987623));
#9080=CARTESIAN_POINT('Ctrl Pts',(0.725288867731711,0.183675686835684,-0.0754012297787415));
#9081=CARTESIAN_POINT('Ctrl Pts',(0.631698822495185,0.201767226924317,0.362657949057064));
#9082=CARTESIAN_POINT('Ctrl Pts',(0.300308325987629,0.219836949162313,0.662675815052713));
#9083=CARTESIAN_POINT('Ctrl Pts',(-0.143562158262448,0.237886151027376,
0.712267282797029));
#9084=CARTESIAN_POINT('Ctrl Pts',(-0.53199081656655,0.255911794003117,0.493667448281364));
#9085=CARTESIAN_POINT('Ctrl Pts',(-0.719417883604853,0.273913307071238,
0.0887760590256471));
#9086=CARTESIAN_POINT('Ctrl Pts',(-0.643660400053528,0.289891600721182,
-0.298017275867573));
#9087=CARTESIAN_POINT('Ctrl Pts',(-0.361885010363615,0.30784406213564,-0.627666996846731));
#9088=CARTESIAN_POINT('Ctrl Pts',(0.0842417800773362,0.325768011230139,
-0.734653870518568));
#9089=CARTESIAN_POINT('Ctrl Pts',(0.517792745159868,0.345644945040527,-0.499418060334344));
#9090=CARTESIAN_POINT('Ctrl Pts',(0.733800619596213,0.365486255885401,-0.0594459732028802));
#9091=CARTESIAN_POINT('Ctrl Pts',(0.582673221392261,0.387265364391542,0.480796666749224));
#9092=CARTESIAN_POINT('Ctrl Pts',(0.0980556067817179,0.408328917576356,
0.719856122275624));
#9093=CARTESIAN_POINT('Ctrl Pts',(-0.340801028355373,0.426717108826706,
0.615863970111398));
#9094=CARTESIAN_POINT('Ctrl Pts',(-0.612394281678541,0.442448812919543,
0.343756687773024));
#9095=CARTESIAN_POINT('Ctrl Pts',(-0.716305141601163,0.460766578913181,
-0.0935336978388081));
#9096=CARTESIAN_POINT('Ctrl Pts',(-0.477493247204526,0.481649255554787,
-0.573041994394618));
#9097=CARTESIAN_POINT('Ctrl Pts',(0.102694969855398,0.505068049619363,-0.736450132310173));
#9098=CARTESIAN_POINT('Ctrl Pts',(0.611261259282936,0.528410394709111,-0.418440438696257));
#9099=CARTESIAN_POINT('Ctrl Pts',(0.718676149949771,0.551673390367526,0.169515917432784));
#9100=CARTESIAN_POINT('Ctrl Pts',(0.356312681653224,0.574854495176515,0.64316080321234));
#9101=CARTESIAN_POINT('Ctrl Pts',(-0.168510516307296,0.595385048110979,
0.688354852013418));
#9102=CARTESIAN_POINT('Ctrl Pts',(-0.528243301677406,0.613292864691495,
0.436029414275985));
#9103=CARTESIAN_POINT('Ctrl Pts',(-0.677381584882317,0.6286030155416,0.0926943249944734));
#9104=CARTESIAN_POINT('Ctrl Pts',(-0.622643305904953,0.643873929815472,
-0.277654803412519));
#9105=CARTESIAN_POINT('Ctrl Pts',(-0.381794378299548,0.65910436568187,-0.562730607759754));
#9106=CARTESIAN_POINT('Ctrl Pts',(-0.028341775812421,0.674293171253774,
-0.677102900368987));
#9107=CARTESIAN_POINT('Ctrl Pts',(0.392731635988073,0.691964896901324,-0.575070914546373));
#9108=CARTESIAN_POINT('Ctrl Pts',(0.69992938794118,0.712091816947967,-0.160128547586193));
#9109=CARTESIAN_POINT('Ctrl Pts',(0.587760439579667,0.734637493639678,0.408855815692916));
#9110=CARTESIAN_POINT('Ctrl Pts',(0.0921415777392107,0.757083566082351,
0.705744227349691));
#9111=CARTESIAN_POINT('Ctrl Pts',(-0.308102004413837,0.773385243522869,
0.585710561547649));
#9112=CARTESIAN_POINT('Ctrl Pts',(-0.478599554075341,0.783594714378652,
0.414507861658026));
#9113=CARTESIAN_POINT('Ctrl Pts',(-0.555934555524573,0.789130340065261,
0.308363588185029));
#9114=CARTESIAN_POINT('Ctrl Pts',(-0.646753984994522,0.799002819487883,
0.0943350303702933));
#9115=CARTESIAN_POINT('Ctrl Pts',(-0.62495936464493,0.809749811628134,-0.179246402023147));
#9116=CARTESIAN_POINT('Ctrl Pts',(-0.491908913808404,0.821352972100955,
-0.404491410613556));
#9117=CARTESIAN_POINT('Ctrl Pts',(-0.362868577423681,0.827552900541956,
-0.515047589824164));
#9118=CARTESIAN_POINT('Ctrl Pts',(-0.250447563309727,0.833262939476477,
-0.574215859282791));
#9119=CARTESIAN_POINT('Ctrl Pts',(-0.134136950448111,0.839898037093364,
-0.613487677738248));
#9120=CARTESIAN_POINT('Ctrl Pts',(0.0314794347668697,0.846658718841028,
-0.627750772072444));
#9121=CARTESIAN_POINT('Ctrl Pts',(0.287859120913106,0.845135120072913,-0.623654695722356));
#9122=CARTESIAN_POINT('Ctrl Pts',(0.544382169584791,0.843101510843351,-0.620927805523985));
#9123=CARTESIAN_POINT('Ctrl Pts',(0.778656772185477,0.844411082457674,-0.62278249525087));
#9124=CARTESIAN_POINT('Ctrl Pts',(1.1044633350947,0.844505710507847,-0.622960502431314));
#9125=CARTESIAN_POINT('Ctrl Pts',(1.51431720637969,0.843878360419051,-0.622011929608527));
#9126=CARTESIAN_POINT('Ctrl Pts',(1.83620514057881,0.844432460340288,-0.622837578949083));
#9127=CARTESIAN_POINT('Ctrl Pts',(2.00012463874466,0.844258347210608,-0.62258250378106));
#9128=CARTESIAN_POINT('Ctrl Pts',(0.665690148929301,0.0540139888223781,
-2.00004484750611));
#9129=CARTESIAN_POINT('Ctrl Pts',(0.6659451150026,0.053839950157021,-1.83619545121158));
#9130=CARTESIAN_POINT('Ctrl Pts',(0.665128143222169,0.0543938477409031,
-1.51455427814217));
#9131=CARTESIAN_POINT('Ctrl Pts',(0.666069495045158,0.0537665346002613,
-1.10412981632951));
#9132=CARTESIAN_POINT('Ctrl Pts',(0.665911310936667,0.0538607932718387,
-0.778993035250902));
#9133=CARTESIAN_POINT('Ctrl Pts',(0.664026136107024,0.0551700417313962,
-0.544470742495059));
#9134=CARTESIAN_POINT('Ctrl Pts',(0.666838914554533,0.0531361927202069,
-0.286662280700477));
#9135=CARTESIAN_POINT('Ctrl Pts',(0.670756199727559,0.0516121409687555,
-0.0329492975889785));
#9136=CARTESIAN_POINT('Ctrl Pts',(0.656928056566985,0.0583614640101509,
0.134122099891118));
#9137=CARTESIAN_POINT('Ctrl Pts',(0.614653651087194,0.0655518749768497,
0.260460791549869));
#9138=CARTESIAN_POINT('Ctrl Pts',(0.550691302932979,0.0716990222856046,
0.381491744797825));
#9139=CARTESIAN_POINT('Ctrl Pts',(0.433937868706107,0.0782551569430249,
0.517766096947181));
#9140=CARTESIAN_POINT('Ctrl Pts',(0.195022227157333,0.0905176840738019,
0.659128805501105));
#9141=CARTESIAN_POINT('Ctrl Pts',(-0.165221803132377,0.104824365687565,
0.686656794439709));
#9142=CARTESIAN_POINT('Ctrl Pts',(-0.575948987297183,0.124434718794426,
0.433851544302891));
#9143=CARTESIAN_POINT('Ctrl Pts',(-0.73284398024972,0.145673674627877,-0.0898275556952109));
#9144=CARTESIAN_POINT('Ctrl Pts',(-0.425082855843943,0.168912723107633,
-0.601402499618176));
#9145=CARTESIAN_POINT('Ctrl Pts',(0.108828702060105,0.19007897377441,-0.706601840568686));
#9146=CARTESIAN_POINT('Ctrl Pts',(0.517997291942158,0.209286498552809,-0.463265327584241));
#9147=CARTESIAN_POINT('Ctrl Pts',(0.689377950201828,0.226516243592352,-0.0734161361504486));
#9148=CARTESIAN_POINT('Ctrl Pts',(0.600353887084564,0.243701687466735,0.342693377829791));
#9149=CARTESIAN_POINT('Ctrl Pts',(0.286030035028936,0.260835983707096,0.627102830068772));
#9150=CARTESIAN_POINT('Ctrl Pts',(-0.134155065157305,0.277920950638178,
0.673933998676897));
#9151=CARTESIAN_POINT('Ctrl Pts',(-0.501164021709181,0.294954365139144,
0.467262210920895));
#9152=CARTESIAN_POINT('Ctrl Pts',(-0.677874728226525,0.311936243936039,
0.0852452309648463));
#9153=CARTESIAN_POINT('Ctrl Pts',(-0.606442919414857,0.326984295200526,
-0.279024712472493));
#9154=CARTESIAN_POINT('Ctrl Pts',(-0.3413638889742,0.343869213947561,-0.589050402985317));
#9155=CARTESIAN_POINT('Ctrl Pts',(0.0776127328996499,0.360700417795057,
-0.689346797344412));
#9156=CARTESIAN_POINT('Ctrl Pts',(0.483925382117204,0.379330610399405,-0.468750804288638));
#9157=CARTESIAN_POINT('Ctrl Pts',(0.685993707862927,0.397899656052825,-0.0569247093507329));
#9158=CARTESIAN_POINT('Ctrl Pts',(0.544593843892337,0.41824532301881,0.447745369014097));
#9159=CARTESIAN_POINT('Ctrl Pts',(0.0926262835585758,0.437885829762225,
0.670478864626929));
#9160=CARTESIAN_POINT('Ctrl Pts',(-0.315940435227643,0.455005455676549,
0.573590148682299));
#9161=CARTESIAN_POINT('Ctrl Pts',(-0.56845556554157,0.469633957922228,0.320516289738299));
#9162=CARTESIAN_POINT('Ctrl Pts',(-0.664899902133018,0.486647192977617,
-0.0856672750405439));
#9163=CARTESIAN_POINT('Ctrl Pts',(-0.443255626672905,0.506013771825995,
-0.530317040586));
#9164=CARTESIAN_POINT('Ctrl Pts',(0.0940211962866315,0.527697344618731,
-0.681439042050755));
#9165=CARTESIAN_POINT('Ctrl Pts',(0.564092381788613,0.549276072844908,-0.387291286681534));
#9166=CARTESIAN_POINT('Ctrl Pts',(0.663088983781026,0.570749464526914,0.155497762155742));
#9167=CARTESIAN_POINT('Ctrl Pts',(0.328929597234121,0.592117299617171,0.592008544234696));
#9168=CARTESIAN_POINT('Ctrl Pts',(-0.154237322206182,0.611016959266645,
0.633500441753773));
#9169=CARTESIAN_POINT('Ctrl Pts',(-0.485035884449274,0.627485653531596,
0.401403084621955));
#9170=CARTESIAN_POINT('Ctrl Pts',(-0.62206334875908,0.641554792618914,0.0858794376383043));
#9171=CARTESIAN_POINT('Ctrl Pts',(-0.571760075942313,0.655576455451205,
-0.254188255862264));
#9172=CARTESIAN_POINT('Ctrl Pts',(-0.350733148500619,0.669551327422222,
-0.51575472245803));
#9173=CARTESIAN_POINT('Ctrl Pts',(-0.0265957997704319,0.683479439931836,
-0.620606617386987));
#9174=CARTESIAN_POINT('Ctrl Pts',(0.35930180280925,0.699674935929321,-0.527065809433042));
#9175=CARTESIAN_POINT('Ctrl Pts',(0.640559927378796,0.718104410331526,-0.147019361766098));
#9176=CARTESIAN_POINT('Ctrl Pts',(0.537831107754837,0.738736997373318,0.373647816694899));
#9177=CARTESIAN_POINT('Ctrl Pts',(0.0845805647471646,0.759259943025514,
0.645113960140173));
#9178=CARTESIAN_POINT('Ctrl Pts',(-0.281268703654681,0.774162449469679,
0.535302832262414));
#9179=CARTESIAN_POINT('Ctrl Pts',(-0.437006958245047,0.783485974077427,
0.378958889142701));
#9180=CARTESIAN_POINT('Ctrl Pts',(-0.507697370885022,0.788549978506264,
0.281850016683051));
#9181=CARTESIAN_POINT('Ctrl Pts',(-0.590811263696918,0.79755702495982,0.0865772474568527));
#9182=CARTESIAN_POINT('Ctrl Pts',(-0.570421542490006,0.807404168621158,
-0.163998512585474));
#9183=CARTESIAN_POINT('Ctrl Pts',(-0.449519165229382,0.817962511928117,
-0.368907152618757));
#9184=CARTESIAN_POINT('Ctrl Pts',(-0.331434707315454,0.823631825677829,
-0.470158335662351));
#9185=CARTESIAN_POINT('Ctrl Pts',(-0.228414168702972,0.828869835105896,
-0.524261354796639));
#9186=CARTESIAN_POINT('Ctrl Pts',(-0.124409789837836,0.83479670994367,-0.559486616067973));
#9187=CARTESIAN_POINT('Ctrl Pts',(0.0311860121700488,0.84127032933758,-0.573462474344531));
#9188=CARTESIAN_POINT('Ctrl Pts',(0.286930207599112,0.839831852204138,-0.56941247728844));
#9189=CARTESIAN_POINT('Ctrl Pts',(0.544368769266695,0.837758405835724,-0.566662924739702));
#9190=CARTESIAN_POINT('Ctrl Pts',(0.77915350747992,0.839083640925069,-0.568525018908883));
#9191=CARTESIAN_POINT('Ctrl Pts',(1.10406134980889,0.839169583354872,-0.568697614612765));
#9192=CARTESIAN_POINT('Ctrl Pts',(1.51463887381527,0.838547420648682,-0.567751119234392));
#9193=CARTESIAN_POINT('Ctrl Pts',(1.83619420925238,0.839098369729373,-0.568574422943627));
#9194=CARTESIAN_POINT('Ctrl Pts',(2.0000345343157,0.838924340696319,-0.568319470976886));
#9195=CARTESIAN_POINT('Ctrl Pts',(0.62672943408441,0.0786682492038075,-1.99995803330129));
#9196=CARTESIAN_POINT('Ctrl Pts',(0.626984281206633,0.0784942917339065,
-1.83618507879303));
#9197=CARTESIAN_POINT('Ctrl Pts',(0.626167881567446,0.0790457108498767,
-1.51485561868953));
#9198=CARTESIAN_POINT('Ctrl Pts',(0.627102473829725,0.0784231080938741,
-1.10373920604851));
#9199=CARTESIAN_POINT('Ctrl Pts',(0.626949240460296,0.0785101683511648,
-0.779449572693693));
#9200=CARTESIAN_POINT('Ctrl Pts',(0.625050745785335,0.0798328338465923,
-0.544462149089626));
#9201=CARTESIAN_POINT('Ctrl Pts',(0.627889985740265,0.0777656623793459,
-0.285696293823589));
#9202=CARTESIAN_POINT('Ctrl Pts',(0.631738128714664,0.0763139712887997,
-0.0328999352935243));
#9203=CARTESIAN_POINT('Ctrl Pts',(0.618203355232202,0.0828217339857707,
0.126016338436061));
#9204=CARTESIAN_POINT('Ctrl Pts',(0.5788696130134,0.089502164873538,0.243540471625212));
#9205=CARTESIAN_POINT('Ctrl Pts',(0.518429935075775,0.0953194797976742,
0.357975889465943));
#9206=CARTESIAN_POINT('Ctrl Pts',(0.4085463000272,0.10148208753481,0.486163680166641));
#9207=CARTESIAN_POINT('Ctrl Pts',(0.18454758337479,0.112981193016189,0.618576938164562));
#9208=CARTESIAN_POINT('Ctrl Pts',(-0.154217959045931,0.126437065904357,
0.644731550026875));
#9209=CARTESIAN_POINT('Ctrl Pts',(-0.53919139895456,0.144820634753371,0.407325706570045));
#9210=CARTESIAN_POINT('Ctrl Pts',(-0.686206851627058,0.164726032742826,
-0.0832228853543702));
#9211=CARTESIAN_POINT('Ctrl Pts',(-0.398055690096881,0.186466555625688,
-0.561844820235381));
#9212=CARTESIAN_POINT('Ctrl Pts',(0.10085458709022,0.206247303003531,-0.659997015644472));
#9213=CARTESIAN_POINT('Ctrl Pts',(0.482784624497038,0.224177467621409,-0.432799283114279));
#9214=CARTESIAN_POINT('Ctrl Pts',(0.642581592200899,0.240248144748989,-0.0691618097941696));
#9215=CARTESIAN_POINT('Ctrl Pts',(0.559567552302235,0.256264600472695,0.318623559236399));
#9216=CARTESIAN_POINT('Ctrl Pts',(0.266823917287717,0.272221182924003,0.583443542472237));
#9217=CARTESIAN_POINT('Ctrl Pts',(-0.124194342342738,0.288120357516062,
0.62698047179839));
#9218=CARTESIAN_POINT('Ctrl Pts',(-0.465474692842472,0.303961011116931,
0.434750176991032));
#9219=CARTESIAN_POINT('Ctrl Pts',(-0.629665991844459,0.319743666769981,
0.0797039890484459));
#9220=CARTESIAN_POINT('Ctrl Pts',(-0.563291828984184,0.333721066643941,
-0.25863406390321));
#9221=CARTESIAN_POINT('Ctrl Pts',(-0.317177505535178,0.349397283704289,
-0.546449972718228));
#9222=CARTESIAN_POINT('Ctrl Pts',(0.0716126775062496,0.365015623748908,
-0.639472176834321));
#9223=CARTESIAN_POINT('Ctrl Pts',(0.44843287350778,0.382294855949406,-0.434852100630385));
#9224=CARTESIAN_POINT('Ctrl Pts',(0.63574682531925,0.399510275598109,-0.0530429731296652));
#9225=CARTESIAN_POINT('Ctrl Pts',(0.504663248626496,0.418366227351729,0.414638002521349));
#9226=CARTESIAN_POINT('Ctrl Pts',(0.0859614245310279,0.436560993262288,
0.620946393148274));
#9227=CARTESIAN_POINT('Ctrl Pts',(-0.292431686101597,0.452416791448528,
0.531200841970267));
#9228=CARTESIAN_POINT('Ctrl Pts',(-0.526265761537412,0.465963442852263,
0.29684552061805));
#9229=CARTESIAN_POINT('Ctrl Pts',(-0.615560796465379,0.481716911656766,
-0.0792565511246861));
#9230=CARTESIAN_POINT('Ctrl Pts',(-0.410344088232626,0.499648879780982,
-0.490947805481661));
#9231=CARTESIAN_POINT('Ctrl Pts',(0.0871079884122845,0.519725898932142,
-0.630875565640356));
#9232=CARTESIAN_POINT('Ctrl Pts',(0.522394114004133,0.539708055100366,-0.35851478036304));
#9233=CARTESIAN_POINT('Ctrl Pts',(0.614106517526869,0.55959700282496,0.144195500945888));
#9234=CARTESIAN_POINT('Ctrl Pts',(0.304551390300492,0.57939424257321,0.548632718489485));
#9235=CARTESIAN_POINT('Ctrl Pts',(-0.143262545090784,0.596911693363567,
0.587123558035457));
#9236=CARTESIAN_POINT('Ctrl Pts',(-0.450004619985209,0.612182310173313,
0.371935416025931));
#9237=CARTESIAN_POINT('Ctrl Pts',(-0.577120807453118,0.62523280671009,0.079266601333838));
#9238=CARTESIAN_POINT('Ctrl Pts',(-0.530462301562817,0.638245507692561,
-0.236320918010667));
#9239=CARTESIAN_POINT('Ctrl Pts',(-0.32526663056702,0.651220933950828,-0.479186888619294));
#9240=CARTESIAN_POINT('Ctrl Pts',(-0.0241756368245449,0.66415927198707,
-0.576609424925001));
#9241=CARTESIAN_POINT('Ctrl Pts',(0.334495973140524,0.679212452857298,-0.489701096053415));
#9242=CARTESIAN_POINT('Ctrl Pts',(0.596200424927635,0.696356179648218,-0.136231806846881));
#9243=CARTESIAN_POINT('Ctrl Pts',(0.500642690062709,0.715568736684096,0.348576033177884));
#9244=CARTESIAN_POINT('Ctrl Pts',(0.0782134587988113,0.734699394529406,
0.601783229446777));
#9245=CARTESIAN_POINT('Ctrl Pts',(-0.263334440263774,0.74861335220138,0.499309887430558));
#9246=CARTESIAN_POINT('Ctrl Pts',(-0.408761144108869,0.75731773364333,0.353356897942407));
#9247=CARTESIAN_POINT('Ctrl Pts',(-0.474830525070825,0.762054113932951,
0.262524775384885));
#9248=CARTESIAN_POINT('Ctrl Pts',(-0.552641913792421,0.770463016151057,
0.0802325505851415));
#9249=CARTESIAN_POINT('Ctrl Pts',(-0.533212125162727,0.779701800604458,
-0.154774313380276));
#9250=CARTESIAN_POINT('Ctrl Pts',(-0.420511229514612,0.789556784600691,
-0.345980730976801));
#9251=CARTESIAN_POINT('Ctrl Pts',(-0.309815844486922,0.794867133309828,
-0.440969276372039));
#9252=CARTESIAN_POINT('Ctrl Pts',(-0.212711168959734,0.799809791402836,
-0.491916344579349));
#9253=CARTESIAN_POINT('Ctrl Pts',(-0.116675449236811,0.805274071611186,
-0.524469634945247));
#9254=CARTESIAN_POINT('Ctrl Pts',(0.0312001431979104,0.811517204070306,
-0.538144006859143));
#9255=CARTESIAN_POINT('Ctrl Pts',(0.285951855836605,0.810147186315183,-0.534168979189779));
#9256=CARTESIAN_POINT('Ctrl Pts',(0.544362350217127,0.808042230889924,-0.531389671259308));
#9257=CARTESIAN_POINT('Ctrl Pts',(0.77960272849961,0.809380172550063,-0.533265960326483));
#9258=CARTESIAN_POINT('Ctrl Pts',(1.10367239586754,0.80945930366762,-0.533432761018123));
#9259=CARTESIAN_POINT('Ctrl Pts',(1.51493665542971,0.808841636111715,-0.532492980025066));
#9260=CARTESIAN_POINT('Ctrl Pts',(1.83618388576743,0.809390251128783,-0.533315228872414));
#9261=CARTESIAN_POINT('Ctrl Pts',(1.99994811217411,0.809216302926719,-0.53306039532281));
#9262=CARTESIAN_POINT('Ctrl Pts',(0.5874609188711,0.0822019824159158,-1.99989317407337));
#9263=CARTESIAN_POINT('Ctrl Pts',(0.587715677265367,0.0820280855113077,
-1.83617723900198));
#9264=CARTESIAN_POINT('Ctrl Pts',(0.58689971250081,0.0825772844454769,-1.51508654260829));
#9265=CARTESIAN_POINT('Ctrl Pts',(0.587831000225384,0.0819585874321892,
-1.10344749883076));
#9266=CARTESIAN_POINT('Ctrl Pts',(0.587680460234937,0.0820393800455694,
-0.779804611248477));
#9267=CARTESIAN_POINT('Ctrl Pts',(0.585775499994469,0.083373568561431,-0.544448425778546));
#9268=CARTESIAN_POINT('Ctrl Pts',(0.58862845690685,0.0812774489656124,-0.285022784695781));
#9269=CARTESIAN_POINT('Ctrl Pts',(0.592441914962544,0.079888127716253,-0.0326774653733658));
#9270=CARTESIAN_POINT('Ctrl Pts',(0.579108229824713,0.086188207924076,0.11900070157323));
#9271=CARTESIAN_POINT('Ctrl Pts',(0.542704406423502,0.0923562996112714,
0.227612687921699));
#9272=CARTESIAN_POINT('Ctrl Pts',(0.485928138725982,0.0978317117759704,
0.335239816192948));
#9273=CARTESIAN_POINT('Ctrl Pts',(0.382789952176369,0.103609371928733,0.455495129550219));
#9274=CARTESIAN_POINT('Ctrl Pts',(0.173445112617297,0.114358088999672,0.579131350820057));
#9275=CARTESIAN_POINT('Ctrl Pts',(-0.144342710046836,0.126982880344674,
0.603964833450006));
#9276=CARTESIAN_POINT('Ctrl Pts',(-0.504617540795482,0.144187615680568,
0.381427965458317));
#9277=CARTESIAN_POINT('Ctrl Pts',(-0.642383911453795,0.162830042168221,
-0.0777436199891682));
#9278=CARTESIAN_POINT('Ctrl Pts',(-0.372578271513367,0.18317769756345,-0.525811039595045));
#9279=CARTESIAN_POINT('Ctrl Pts',(0.0943497013842308,0.201692512692434,
-0.617644888618581));
#9280=CARTESIAN_POINT('Ctrl Pts',(0.451815269396865,0.218473010441523,-0.405014599643461));
#9281=CARTESIAN_POINT('Ctrl Pts',(0.601373785637953,0.233514060494329,-0.0646699181159046));
#9282=CARTESIAN_POINT('Ctrl Pts',(0.523679013910274,0.248505254417583,0.29829880585065));
#9283=CARTESIAN_POINT('Ctrl Pts',(0.24964403741173,0.263442115335976,0.546206089476511));
#9284=CARTESIAN_POINT('Ctrl Pts',(-0.116451337731323,0.278327625975953,
0.586979022297046));
#9285=CARTESIAN_POINT('Ctrl Pts',(-0.436054891647266,0.29316158596241,0.406974772591184));
#9286=CARTESIAN_POINT('Ctrl Pts',(-0.589870298345399,0.30794504129165,0.0744078582288452));
#9287=CARTESIAN_POINT('Ctrl Pts',(-0.527692943172682,0.321041534993931,
-0.242618792914012));
#9288=CARTESIAN_POINT('Ctrl Pts',(-0.297023701829149,0.335734465321562,
-0.512391077873751));
#9289=CARTESIAN_POINT('Ctrl Pts',(0.0675212641741527,0.35037904755484,-0.5996538147588));
#9290=CARTESIAN_POINT('Ctrl Pts',(0.421056594556602,0.366589258750743,-0.407716742702501));
#9291=CARTESIAN_POINT('Ctrl Pts',(0.596905393478329,0.382748228505995,-0.0493501504687293));
#9292=CARTESIAN_POINT('Ctrl Pts',(0.473862910947153,0.400458116239252,0.389940683934648));
#9293=CARTESIAN_POINT('Ctrl Pts',(0.0802903162289862,0.417561901608528,
0.583953158059964));
#9294=CARTESIAN_POINT('Ctrl Pts',(-0.275709966682282,0.432478726710855,
0.499557870740994));
#9295=CARTESIAN_POINT('Ctrl Pts',(-0.495862448390292,0.445231474030675,
0.278949853677765));
#9296=CARTESIAN_POINT('Ctrl Pts',(-0.580023400465553,0.46007217823348,-0.0753512915820435));
#9297=CARTESIAN_POINT('Ctrl Pts',(-0.386607022200923,0.476980336558612,
-0.463591036362349));
#9298=CARTESIAN_POINT('Ctrl Pts',(0.0829877251595423,0.495934135576676,
-0.595818995283933));
#9299=CARTESIAN_POINT('Ctrl Pts',(0.494534882711716,0.514822618485088,-0.338472445755909));
#9300=CARTESIAN_POINT('Ctrl Pts',(0.581491499979929,0.533648931251995,0.137363743733339));
#9301=CARTESIAN_POINT('Ctrl Pts',(0.288161264391336,0.552415905203638,0.52085580206473));
#9302=CARTESIAN_POINT('Ctrl Pts',(-0.137003162728498,0.569047439534844,
0.557541558510368));
#9303=CARTESIAN_POINT('Ctrl Pts',(-0.428676822886062,0.583565633440864,
0.352995905254951));
#9304=CARTESIAN_POINT('Ctrl Pts',(-0.549711004700905,0.595987212241011,
0.0744483287800028));
#9305=CARTESIAN_POINT('Ctrl Pts',(-0.505299948228852,0.608386728377244,
-0.226282687840735));
#9306=CARTESIAN_POINT('Ctrl Pts',(-0.309575039133742,0.620765578833677,
-0.45802323172802));
#9307=CARTESIAN_POINT('Ctrl Pts',(-0.0219755772339618,0.633124488893754,
-0.551129760420029));
#9308=CARTESIAN_POINT('Ctrl Pts',(0.321081796479251,0.647521942421836,-0.468075339341517));
#9309=CARTESIAN_POINT('Ctrl Pts',(0.571917008721482,0.663944142090889,-0.129561094078861));
#9310=CARTESIAN_POINT('Ctrl Pts',(0.480393018973127,0.682387090247801,0.335843108412934));
#9311=CARTESIAN_POINT('Ctrl Pts',(0.0741693531238315,0.700787378825874,
0.57961025567971));
#9312=CARTESIAN_POINT('Ctrl Pts',(-0.255143275996557,0.714201786052559,
0.480937271720544));
#9313=CARTESIAN_POINT('Ctrl Pts',(-0.395498171738189,0.722601182697331,
0.340100684060336));
#9314=CARTESIAN_POINT('Ctrl Pts',(-0.459314101410141,0.727177877012928,
0.252326763909831));
#9315=CARTESIAN_POINT('Ctrl Pts',(-0.534583243568393,0.735297491050186,
0.0763204025504257));
#9316=CARTESIAN_POINT('Ctrl Pts',(-0.515616512133595,0.7442503799837,-0.151391320167515));
#9317=CARTESIAN_POINT('Ctrl Pts',(-0.406711704651741,0.753781299451576,
-0.336277015933739));
#9318=CARTESIAN_POINT('Ctrl Pts',(-0.299435189638348,0.758923960221984,
-0.428370572052981));
#9319=CARTESIAN_POINT('Ctrl Pts',(-0.204694398152886,0.763750096791064,
-0.47808447397292));
#9320=CARTESIAN_POINT('Ctrl Pts',(-0.112050112984815,0.769013820539994,
-0.509451539857503));
#9321=CARTESIAN_POINT('Ctrl Pts',(0.0314195100887834,0.775117938261012,
-0.522885083062355));
#9322=CARTESIAN_POINT('Ctrl Pts',(0.285217271752917,0.773788624023985,-0.518977616945277));
#9323=CARTESIAN_POINT('Ctrl Pts',(0.544377275887181,0.7716647254831,-0.516167687470469));
#9324=CARTESIAN_POINT('Ctrl Pts',(0.77992084130335,0.773010147661079,-0.518055833052231));
#9325=CARTESIAN_POINT('Ctrl Pts',(1.10339956738025,0.773085111411238,-0.518215860268804));
#9326=CARTESIAN_POINT('Ctrl Pts',(1.51514747628628,0.772470044939352,-0.517280005423198));
#9327=CARTESIAN_POINT('Ctrl Pts',(1.83617635170566,0.773017182662106,-0.518099756538723));
#9328=CARTESIAN_POINT('Ctrl Pts',(1.99988580057488,0.77284329264402,-0.517845008228458));
#9329=CARTESIAN_POINT('Ctrl Pts',(0.550945450866199,0.067105092762305,-1.99985238806428));
#9330=CARTESIAN_POINT('Ctrl Pts',(0.551200153361326,0.0669312340141922,
-1.83617237557771));
#9331=CARTESIAN_POINT('Ctrl Pts',(0.550383059047253,0.067478738759276,-1.51523700162691));
#9332=CARTESIAN_POINT('Ctrl Pts',(0.551312121940096,0.0668631648982134,
-1.10325776056893));
#9333=CARTESIAN_POINT('Ctrl Pts',(0.551160834485697,0.0669390897119991,
-0.780037484764116));
#9334=CARTESIAN_POINT('Ctrl Pts',(0.549254306488641,0.0682824421640895,
-0.544421315854621));
#9335=CARTESIAN_POINT('Ctrl Pts',(0.552106416364749,0.0661635755354553,
-0.284639224380358));
#9336=CARTESIAN_POINT('Ctrl Pts',(0.555914749094926,0.0648235660252144,
-0.0323032591833498));
#9337=CARTESIAN_POINT('Ctrl Pts',(0.542682333476631,0.0709613521230218,
0.11348170634836));
#9338=CARTESIAN_POINT('Ctrl Pts',(0.508977099615909,0.0766537088572853,
0.213768678876433));
#9339=CARTESIAN_POINT('Ctrl Pts',(0.455708834950571,0.0818026163180467,
0.314916823094266));
#9340=CARTESIAN_POINT('Ctrl Pts',(0.358692386569373,0.0872323354600932,
0.427975224214404));
#9341=CARTESIAN_POINT('Ctrl Pts',(0.162663694190769,0.097298924680809,0.543646775182899));
#9342=CARTESIAN_POINT('Ctrl Pts',(-0.136192113262965,0.109174509901586,
0.567305343826758));
#9343=CARTESIAN_POINT('Ctrl Pts',(-0.474558443064967,0.125332340697949,
0.358045956782264));
#9344=CARTESIAN_POINT('Ctrl Pts',(-0.60433801784961,0.142871565376813,-0.0736684299162183));
#9345=CARTESIAN_POINT('Ctrl Pts',(-0.350381954033981,0.162024342912799,
-0.495576784770102));
#9346=CARTESIAN_POINT('Ctrl Pts',(0.0896117759143228,0.179474692463962,
-0.582204390142572));
#9347=CARTESIAN_POINT('Ctrl Pts',(0.426885853840544,0.195305136977579,-0.381668836262442));
#9348=CARTESIAN_POINT('Ctrl Pts',(0.568149223251883,0.20950819707601,-0.0603124683763491));
#9349=CARTESIAN_POINT('Ctrl Pts',(0.494770009110161,0.22367796540124,0.282770658933988));
#9350=CARTESIAN_POINT('Ctrl Pts',(0.235528087739685,0.237810882245137,0.517373264212428));
#9351=CARTESIAN_POINT('Ctrl Pts',(-0.111222533228894,0.251910335567996,
0.556051654550424));
#9352=CARTESIAN_POINT('Ctrl Pts',(-0.414313232539064,0.265976879461039,
0.385418487215813));
#9353=CARTESIAN_POINT('Ctrl Pts',(-0.560401318983622,0.280011870110238,
0.0697231995474879));
#9354=CARTESIAN_POINT('Ctrl Pts',(-0.501352286024681,0.292460599828054,
-0.231630199439596));
#9355=CARTESIAN_POINT('Ctrl Pts',(-0.281902903004944,0.306441274341836,
-0.488339555795956));
#9356=CARTESIAN_POINT('Ctrl Pts',(0.065387266285567,0.320393957968718,-0.571596489894968));
#9357=CARTESIAN_POINT('Ctrl Pts',(0.402799127650896,0.335863029162657,-0.388516285439416));
#9358=CARTESIAN_POINT('Ctrl Pts',(0.570909994761135,0.351304546428848,-0.0461096493466856));
#9359=CARTESIAN_POINT('Ctrl Pts',(0.453309975606592,0.368257239503034,0.374426206306753));
#9360=CARTESIAN_POINT('Ctrl Pts',(0.0759001441926504,0.384661798048627,
0.560666086673735));
#9361=CARTESIAN_POINT('Ctrl Pts',(-0.266151455502317,0.398993403813706,
0.479651913020883));
#9362=CARTESIAN_POINT('Ctrl Pts',(-0.478001702726463,0.411263096833331,
0.267441030022521));
#9363=CARTESIAN_POINT('Ctrl Pts',(-0.55916305232678,0.425562184968444,-0.0738989456599627));
#9364=CARTESIAN_POINT('Ctrl Pts',(-0.372636699601196,0.441883583112284,
-0.448734050354975));
#9365=CARTESIAN_POINT('Ctrl Pts',(0.0816035926774441,0.460220680465181,
-0.576880646792149));
#9366=CARTESIAN_POINT('Ctrl Pts',(0.480801224099281,0.478537007133273,-0.327530135042584));
#9367=CARTESIAN_POINT('Ctrl Pts',(0.565551782967983,0.496836451246379,0.134930498293982));
#9368=CARTESIAN_POINT('Ctrl Pts',(0.279939442908263,0.515122401597484,0.508738501339385));
#9369=CARTESIAN_POINT('Ctrl Pts',(-0.135321607217399,0.5313675615131,0.544776075890801));
#9370=CARTESIAN_POINT('Ctrl Pts',(-0.420872324450394,0.54557805985139,0.344637404158902));
#9371=CARTESIAN_POINT('Ctrl Pts',(-0.539596413905804,0.557756821355681,
0.071564075139448));
#9372=CARTESIAN_POINT('Ctrl Pts',(-0.496054610193741,0.569935034483373,
-0.223801635132005));
#9373=CARTESIAN_POINT('Ctrl Pts',(-0.303551962745066,0.582113820788074,
-0.451841305044243));
#9374=CARTESIAN_POINT('Ctrl Pts',(-0.0201376858984327,0.594293856531097,
-0.543665136012608));
#9375=CARTESIAN_POINT('Ctrl Pts',(0.318550684880049,0.608507626299889,-0.461760947931387));
#9376=CARTESIAN_POINT('Ctrl Pts',(0.56690994352398,0.624756550847024,-0.126963600293733));
#9377=CARTESIAN_POINT('Ctrl Pts',(0.47637525653217,0.643052724327624,0.334766757063998));
#9378=CARTESIAN_POINT('Ctrl Pts',(0.0724483648226123,0.661355498523464,
0.577485257188254));
#9379=CARTESIAN_POINT('Ctrl Pts',(-0.256055153330988,0.674735290731573,
0.479237459957281));
#9380=CARTESIAN_POINT('Ctrl Pts',(-0.396261391483261,0.683125208503875,
0.338563008491415));
#9381=CARTESIAN_POINT('Ctrl Pts',(-0.460044070922385,0.687699882890572,
0.250826790073639));
#9382=CARTESIAN_POINT('Ctrl Pts',(-0.535356310780212,0.695820111538706,
0.0748271639382049));
#9383=CARTESIAN_POINT('Ctrl Pts',(-0.51637969164712,0.704791213538561,-0.153359389343171));
#9384=CARTESIAN_POINT('Ctrl Pts',(-0.407166121656258,0.714351503734276,
-0.338801256616131));
#9385=CARTESIAN_POINT('Ctrl Pts',(-0.299604806090809,0.7195056868629,-0.431148288532543));
#9386=CARTESIAN_POINT('Ctrl Pts',(-0.20397209222849,0.724379105857744,-0.481389271359994));
#9387=CARTESIAN_POINT('Ctrl Pts',(-0.110498436078102,0.729684445910484,
-0.512948589891693));
#9388=CARTESIAN_POINT('Ctrl Pts',(0.0317754025745838,0.73573981334391,-0.526218953561026));
#9389=CARTESIAN_POINT('Ctrl Pts',(0.284730439464858,0.734424495251457,-0.522371841874736));
#9390=CARTESIAN_POINT('Ctrl Pts',(0.544396269643961,0.732294283957779,-0.519536512654844));
#9391=CARTESIAN_POINT('Ctrl Pts',(0.780091402972714,0.73364230094729,-0.521435851662876));
#9392=CARTESIAN_POINT('Ctrl Pts',(1.10324034467337,0.733715868350949,-0.521590658029006));
#9393=CARTESIAN_POINT('Ctrl Pts',(1.51526428502092,0.733101852305696,-0.520659208592313));
#9394=CARTESIAN_POINT('Ctrl Pts',(1.83617199619976,0.73364855145534,-0.521477483502039));
#9395=CARTESIAN_POINT('Ctrl Pts',(1.9998492399299,0.733474695645128,-0.521222785306198));
#9396=CARTESIAN_POINT('Ctrl Pts',(0.534004674862244,0.0469900053766836,
-1.99984739250011));
#9397=CARTESIAN_POINT('Ctrl Pts',(0.534259370517448,0.0468161512974708,
-1.83617177556803));
#9398=CARTESIAN_POINT('Ctrl Pts',(0.533441502311306,0.047363056988596,-1.51526191633464));
#9399=CARTESIAN_POINT('Ctrl Pts',(0.534371434639262,0.0467484424255759,
-1.10323146349633));
#9400=CARTESIAN_POINT('Ctrl Pts',(0.53421824455692,0.0468227288278506,-0.780080082057997));
#9401=CARTESIAN_POINT('Ctrl Pts',(0.53231508003366,0.0481691265924268,-0.5444042631695));
#9402=CARTESIAN_POINT('Ctrl Pts',(0.53515856794429,0.0460425754822485,-0.284643294266451));
#9403=CARTESIAN_POINT('Ctrl Pts',(0.538985648847748,0.0447190117196379,
-0.0320211294696051));
#9404=CARTESIAN_POINT('Ctrl Pts',(0.525741686811735,0.0508034693757587,
0.111631344947843));
#9405=CARTESIAN_POINT('Ctrl Pts',(0.493267866324073,0.0562760720192935,
0.208037659421039));
#9406=CARTESIAN_POINT('Ctrl Pts',(0.441696713730458,0.0612676600297227,
0.306080548947707));
#9407=CARTESIAN_POINT('Ctrl Pts',(0.347410886319535,0.0665431383971926,
0.415933050789519));
#9408=CARTESIAN_POINT('Ctrl Pts',(0.157327861273452,0.0763049024739723,
0.528057489188086));
#9409=CARTESIAN_POINT('Ctrl Pts',(-0.133156674943477,0.0878492851954371,
0.551209324434459));
#9410=CARTESIAN_POINT('Ctrl Pts',(-0.462129068607569,0.103556824422786,
0.347710166812253));
#9411=CARTESIAN_POINT('Ctrl Pts',(-0.588638599629634,0.120634315916664,
-0.0725030008931035));
#9412=CARTESIAN_POINT('Ctrl Pts',(-0.341164585828511,0.139304871497971,
-0.483904151910011));
#9413=CARTESIAN_POINT('Ctrl Pts',(0.0883544884891012,0.15634168137637,-0.568597044331401));
#9414=CARTESIAN_POINT('Ctrl Pts',(0.418095753693205,0.171816150349456,-0.372629793275881));
#9415=CARTESIAN_POINT('Ctrl Pts',(0.556391570690854,0.185715675527505,-0.0581644462312985));
#9416=CARTESIAN_POINT('Ctrl Pts',(0.484561146319725,0.199598451089136,0.277982796567569));
#9417=CARTESIAN_POINT('Ctrl Pts',(0.230314847899877,0.213461297531163,0.508150230707778));
#9418=CARTESIAN_POINT('Ctrl Pts',(-0.110207364221293,0.227307713902608,
0.546197798579722));
#9419=CARTESIAN_POINT('Ctrl Pts',(-0.408248667614897,0.241138498233169,
0.378481405677519));
#9420=CARTESIAN_POINT('Ctrl Pts',(-0.55212786122253,0.254955114808116,0.0677253194967843));
#9421=CARTESIAN_POINT('Ctrl Pts',(-0.493976322541745,0.267225343790709,
-0.229320675962668));
#9422=CARTESIAN_POINT('Ctrl Pts',(-0.277480263691582,0.281019977096165,
-0.482633192044066));
#9423=CARTESIAN_POINT('Ctrl Pts',(0.065596463336222,0.294804411465538,-0.564997000764067));
#9424=CARTESIAN_POINT('Ctrl Pts',(0.399482932950473,0.310109780450929,-0.38392530822993));
#9425=CARTESIAN_POINT('Ctrl Pts',(0.56609494129569,0.325407661924638,-0.0447422502843249));
#9426=CARTESIAN_POINT('Ctrl Pts',(0.449568840578391,0.342228227329634,0.372555088313464));
#9427=CARTESIAN_POINT('Ctrl Pts',(0.0745015920546068,0.358533475231174,
0.557805153430069));
#9428=CARTESIAN_POINT('Ctrl Pts',(-0.265999568209032,0.372799304426681,
0.477222072678098));
#9429=CARTESIAN_POINT('Ctrl Pts',(-0.477158534899731,0.385027113765151,
0.265766140699257));
#9430=CARTESIAN_POINT('Ctrl Pts',(-0.55819880007667,0.399294294380163,-0.0747901036973868));
#9431=CARTESIAN_POINT('Ctrl Pts',(-0.371948198635926,0.41560348526982,-0.4494077686762));
#9432=CARTESIAN_POINT('Ctrl Pts',(0.0827104291202138,0.433959582494683,
-0.577860783198243));
#9433=CARTESIAN_POINT('Ctrl Pts',(0.483129998632293,0.452327631229365,-0.327955043863337));
#9434=CARTESIAN_POINT('Ctrl Pts',(0.568442679422367,0.47071146405326,0.13660223562247));
#9435=CARTESIAN_POINT('Ctrl Pts',(0.281144892082092,0.489114336526312,0.51291059653611));
#9436=CARTESIAN_POINT('Ctrl Pts',(-0.137494533186177,0.50549224525999,0.549390016718285));
#9437=CARTESIAN_POINT('Ctrl Pts',(-0.425840925255912,0.519839749453121,
0.347369191128545));
#9438=CARTESIAN_POINT('Ctrl Pts',(-0.545888211304912,0.53215017858499,0.0713630548919239));
#9439=CARTESIAN_POINT('Ctrl Pts',(-0.50187537147456,0.544474304440711,-0.227546071152447));
#9440=CARTESIAN_POINT('Ctrl Pts',(-0.306881264535124,0.556813096530318,
-0.458613263717583));
#9441=CARTESIAN_POINT('Ctrl Pts',(-0.0194326697730112,0.569167100060671,
-0.551791152038062));
#9442=CARTESIAN_POINT('Ctrl Pts',(0.324485383771089,0.583600014619787,-0.46868203399731));
#9443=CARTESIAN_POINT('Ctrl Pts',(0.57713540063447,0.600122698894204,-0.12833611767096));
#9444=CARTESIAN_POINT('Ctrl Pts',(0.485092061602979,0.618757114787167,0.341960480204146));
#9445=CARTESIAN_POINT('Ctrl Pts',(0.0731066834054238,0.637429046052168,
0.589705029297371));
#9446=CARTESIAN_POINT('Ctrl Pts',(-0.262559945489057,0.651098951528179,
0.489439247431335));
#9447=CARTESIAN_POINT('Ctrl Pts',(-0.40596163751793,0.659680303032932,0.345554732462302));
#9448=CARTESIAN_POINT('Ctrl Pts',(-0.47120314927041,0.664358692530949,0.255830744517815));
#9449=CARTESIAN_POINT('Ctrl Pts',(-0.548255068766781,0.672671758647096,
0.0756627500398241));
#9450=CARTESIAN_POINT('Ctrl Pts',(-0.528961115138206,0.681853354797658,
-0.157915933389433));
#9451=CARTESIAN_POINT('Ctrl Pts',(-0.41686144719521,0.691663500854672,-0.348212222865038));
#9452=CARTESIAN_POINT('Ctrl Pts',(-0.306694249169893,0.696942448975099,
-0.442778117175704));
#9453=CARTESIAN_POINT('Ctrl Pts',(-0.208440137034481,0.701948967530146,
-0.494458985485184));
#9454=CARTESIAN_POINT('Ctrl Pts',(-0.111735576307102,0.707436605013493,
-0.527032573056622));
#9455=CARTESIAN_POINT('Ctrl Pts',(0.0320564404187695,0.713526797401297,
-0.540268761905287));
#9456=CARTESIAN_POINT('Ctrl Pts',(0.284651256534309,0.712200783188229,-0.53644652612564));
#9457=CARTESIAN_POINT('Ctrl Pts',(0.544412867618483,0.710075632452311,-0.533600539455794));
#9458=CARTESIAN_POINT('Ctrl Pts',(0.780083942590528,0.711421670395101,-0.535504501896504));
#9459=CARTESIAN_POINT('Ctrl Pts',(1.10323653929954,0.711496312658999,-0.535657095037923));
#9460=CARTESIAN_POINT('Ctrl Pts',(1.51526257912182,0.710881717500948,-0.534727266050874));
#9461=CARTESIAN_POINT('Ctrl Pts',(1.83617179277114,0.711428825678065,-0.535544837400977));
#9462=CARTESIAN_POINT('Ctrl Pts',(1.99984752864807,0.711254971469475,-0.535290141551507));
#9463=CARTESIAN_POINT('Ctrl Pts',(0.528325516000818,0.0355351383793534,
-1.99985072236852));
#9464=CARTESIAN_POINT('Ctrl Pts',(0.528580216238454,0.0353612811721935,
-1.83617216061816));
#9465=CARTESIAN_POINT('Ctrl Pts',(0.527761919981528,0.0359080598807752,
-1.51525401386864));
#9466=CARTESIAN_POINT('Ctrl Pts',(0.528692709166738,0.0352936010092843,
-1.10324464383216));
#9467=CARTESIAN_POINT('Ctrl Pts',(0.528538249039279,0.0353675670609071,
-0.780070492797932));
#9468=CARTESIAN_POINT('Ctrl Pts',(0.526637602108816,0.0367145593105412,
-0.544396520018928));
#9469=CARTESIAN_POINT('Ctrl Pts',(0.529475094326102,0.0345864750367511,
-0.284709647833573));
#9470=CARTESIAN_POINT('Ctrl Pts',(0.533315915563189,0.0332661260171643,
-0.0318866342588667));
#9471=CARTESIAN_POINT('Ctrl Pts',(0.520046729613095,0.0393406257213133,
0.111267345674666));
#9472=CARTESIAN_POINT('Ctrl Pts',(0.487978555806356,0.0447398499197174,
0.206365118213754));
#9473=CARTESIAN_POINT('Ctrl Pts',(0.437001774418032,0.0496765590551313,
0.303330442803063));
#9474=CARTESIAN_POINT('Ctrl Pts',(0.34359217210679,0.054902908379379,0.412155588816351));
#9475=CARTESIAN_POINT('Ctrl Pts',(0.155419901809077,0.064566620841489,0.523143450471739));
#9476=CARTESIAN_POINT('Ctrl Pts',(-0.132406193515106,0.076005890905876,
0.5461393872929));
#9477=CARTESIAN_POINT('Ctrl Pts',(-0.4585052544005,0.0915751768415844,0.344428446786955));
#9478=CARTESIAN_POINT('Ctrl Pts',(-0.584075679141621,0.108515922097861,
-0.0723729196787201));
#9479=CARTESIAN_POINT('Ctrl Pts',(-0.338462248411882,0.12705070506418,-0.480836123882888));
#9480=CARTESIAN_POINT('Ctrl Pts',(0.0882708030427006,0.143977745088325,
-0.565053420420048));
#9481=CARTESIAN_POINT('Ctrl Pts',(0.416146086422155,0.159363348118548,-0.370243292897184));
#9482=CARTESIAN_POINT('Ctrl Pts',(0.553763732742827,0.173191747342348,-0.0573989645046387));
#9483=CARTESIAN_POINT('Ctrl Pts',(0.482289890064134,0.18701212633461,0.277245974053173));
#9484=CARTESIAN_POINT('Ctrl Pts',(0.229047329307677,0.200821415024854,0.506551175681503));
#9485=CARTESIAN_POINT('Ctrl Pts',(-0.110374003483933,0.214623123412753,
0.544510067179701));
#9486=CARTESIAN_POINT('Ctrl Pts',(-0.40766150283296,0.228418090582837,0.377257404939042));
#9487=CARTESIAN_POINT('Ctrl Pts',(-0.551295150396298,0.242207808252135,
0.0671188908067961));
#9488=CARTESIAN_POINT('Ctrl Pts',(-0.493245643443692,0.254462036591453,
-0.229548648448914));
#9489=CARTESIAN_POINT('Ctrl Pts',(-0.276929936242163,0.268246205655378,
-0.48268043415828));
#9490=CARTESIAN_POINT('Ctrl Pts',(0.0660979817878402,0.282029157249401,
-0.56509208661935));
#9491=CARTESIAN_POINT('Ctrl Pts',(0.400224908210924,0.297344357665888,-0.383938719179592));
#9492=CARTESIAN_POINT('Ctrl Pts',(0.567086603737135,0.312662109365757,-0.0443326451316622));
#9493=CARTESIAN_POINT('Ctrl Pts',(0.450399697790572,0.329517044874313,0.373843214320543));
#9494=CARTESIAN_POINT('Ctrl Pts',(0.0742631586112486,0.34586991722832,0.559702372303342));
#9495=CARTESIAN_POINT('Ctrl Pts',(-0.267488833499262,0.360187667101961,
0.478855140322724));
#9496=CARTESIAN_POINT('Ctrl Pts',(-0.479552956006764,0.37246695090628,0.266522113563231));
#9497=CARTESIAN_POINT('Ctrl Pts',(-0.561010089555589,0.386802304605621,
-0.0756527104584505));
#9498=CARTESIAN_POINT('Ctrl Pts',(-0.37380142743242,0.40320076618434,-0.45235567176097));
#9499=CARTESIAN_POINT('Ctrl Pts',(0.0837105500021586,0.421672872730665,
-0.581703055845243));
#9500=CARTESIAN_POINT('Ctrl Pts',(0.487040755149608,0.44017222169388,-0.330077148654899));
#9501=CARTESIAN_POINT('Ctrl Pts',(0.573113162045742,0.458702465869511,0.138170100375564));
#9502=CARTESIAN_POINT('Ctrl Pts',(0.28335615351346,0.477266726235763,0.517831802862951));
#9503=CARTESIAN_POINT('Ctrl Pts',(-0.139284333173075,0.493801248027276,
0.55472840308304));
#9504=CARTESIAN_POINT('Ctrl Pts',(-0.430595948725319,0.508295268527237,
0.350662848554826));
#9505=CARTESIAN_POINT('Ctrl Pts',(-0.551949910444459,0.520737729754399,
0.0717040146871301));
#9506=CARTESIAN_POINT('Ctrl Pts',(-0.507464290067291,0.533200036194741,
-0.230562528994356));
#9507=CARTESIAN_POINT('Ctrl Pts',(-0.31020166413149,0.545683273612848,-0.464351384435429));
#9508=CARTESIAN_POINT('Ctrl Pts',(-0.0192492650129703,0.558188014622219,
-0.558684300589107));
#9509=CARTESIAN_POINT('Ctrl Pts',(0.329035122965687,0.572803913266816,-0.474545710915398));
#9510=CARTESIAN_POINT('Ctrl Pts',(0.585077648306754,0.589545384238961,-0.129724768044979));
#9511=CARTESIAN_POINT('Ctrl Pts',(0.49182251269281,0.608439403717184,0.347142406791056));
#9512=CARTESIAN_POINT('Ctrl Pts',(0.0738519459812565,0.627383860376655,
0.598553246116509));
#9513=CARTESIAN_POINT('Ctrl Pts',(-0.26692557334338,0.641260854247049,0.496816287527571));
#9514=CARTESIAN_POINT('Ctrl Pts',(-0.412574454609541,0.649976893163681,
0.350671912292324));
#9515=CARTESIAN_POINT('Ctrl Pts',(-0.478836302760905,0.654727738162907,
0.259559307243844));
#9516=CARTESIAN_POINT('Ctrl Pts',(-0.557090734433065,0.663174756391869,
0.0764917316856528));
#9517=CARTESIAN_POINT('Ctrl Pts',(-0.537578911396685,0.672499276473955,
-0.160750767756091));
#9518=CARTESIAN_POINT('Ctrl Pts',(-0.423523769730798,0.682478242160259,
-0.354329770148811));
#9519=CARTESIAN_POINT('Ctrl Pts',(-0.311592602102818,0.687841923158427,
-0.450394818907249));
#9520=CARTESIAN_POINT('Ctrl Pts',(-0.211664235020424,0.692933107210186,
-0.502988933683848));
#9521=CARTESIAN_POINT('Ctrl Pts',(-0.11285095039931,0.698540582073528,-0.536235596855463));
#9522=CARTESIAN_POINT('Ctrl Pts',(0.0321957650443905,0.704663061559795,
-0.549474282988733));
#9523=CARTESIAN_POINT('Ctrl Pts',(0.284679981111006,0.70332721476915,-0.545658664585203));
#9524=CARTESIAN_POINT('Ctrl Pts',(0.544423010813361,0.701206594196697,-0.542808989660773));
#9525=CARTESIAN_POINT('Ctrl Pts',(0.780051600334079,0.702550794007654,-0.544713980589938));
#9526=CARTESIAN_POINT('Ctrl Pts',(1.10326148850366,0.702626394058564,-0.544865639596336));
#9527=CARTESIAN_POINT('Ctrl Pts',(1.51524226187871,0.702011181204639,-0.543935752090523));
#9528=CARTESIAN_POINT('Ctrl Pts',(1.83617236681158,0.702558621549799,-0.544752786768393));
#9529=CARTESIAN_POINT('Ctrl Pts',(1.9998524353109,0.702384762739154,-0.544498084176928));
#9530=CARTESIAN_POINT('',(1.9998524353109,0.702384762739154,-0.544498084176928));
#9531=CARTESIAN_POINT('',(0.528325516000818,0.0355351383793534,-1.99985072236852));
#9532=CARTESIAN_POINT('Ctrl Pts',(1.9998524353109,0.702384762739154,-0.544498084176928));
#9533=CARTESIAN_POINT('Ctrl Pts',(1.83617236681158,0.702558621549799,-0.544752786768393));
#9534=CARTESIAN_POINT('Ctrl Pts',(1.51524226187871,0.702011181204639,-0.543935752090523));
#9535=CARTESIAN_POINT('Ctrl Pts',(1.10326148850366,0.702626394058564,-0.544865639596336));
#9536=CARTESIAN_POINT('Ctrl Pts',(0.780051600334079,0.702550794007654,-0.544713980589938));
#9537=CARTESIAN_POINT('Ctrl Pts',(0.544423010813361,0.701206594196697,-0.542808989660773));
#9538=CARTESIAN_POINT('Ctrl Pts',(0.284679981111006,0.70332721476915,-0.545658664585203));
#9539=CARTESIAN_POINT('Ctrl Pts',(0.0321957650443905,0.704663061559795,
-0.549474282988733));
#9540=CARTESIAN_POINT('Ctrl Pts',(-0.11285095039931,0.698540582073528,-0.536235596855463));
#9541=CARTESIAN_POINT('Ctrl Pts',(-0.211664235020424,0.692933107210186,
-0.502988933683848));
#9542=CARTESIAN_POINT('Ctrl Pts',(-0.311592602102818,0.687841923158427,
-0.450394818907249));
#9543=CARTESIAN_POINT('Ctrl Pts',(-0.423523769730798,0.682478242160259,
-0.354329770148811));
#9544=CARTESIAN_POINT('Ctrl Pts',(-0.537578911396685,0.672499276473955,
-0.160750767756091));
#9545=CARTESIAN_POINT('Ctrl Pts',(-0.557090734433065,0.663174756391869,
0.0764917316856528));
#9546=CARTESIAN_POINT('Ctrl Pts',(-0.478836302760905,0.654727738162907,
0.259559307243844));
#9547=CARTESIAN_POINT('Ctrl Pts',(-0.412574454609541,0.649976893163681,
0.350671912292324));
#9548=CARTESIAN_POINT('Ctrl Pts',(-0.26692557334338,0.641260854247049,0.496816287527571));
#9549=CARTESIAN_POINT('Ctrl Pts',(0.0738519459812565,0.627383860376655,
0.598553246116509));
#9550=CARTESIAN_POINT('Ctrl Pts',(0.49182251269281,0.608439403717184,0.347142406791056));
#9551=CARTESIAN_POINT('Ctrl Pts',(0.585077648306754,0.589545384238961,-0.129724768044979));
#9552=CARTESIAN_POINT('Ctrl Pts',(0.329035122965687,0.572803913266816,-0.474545710915398));
#9553=CARTESIAN_POINT('Ctrl Pts',(-0.0192492650129703,0.558188014622219,
-0.558684300589107));
#9554=CARTESIAN_POINT('Ctrl Pts',(-0.31020166413149,0.545683273612848,-0.464351384435429));
#9555=CARTESIAN_POINT('Ctrl Pts',(-0.507464290067291,0.533200036194741,
-0.230562528994356));
#9556=CARTESIAN_POINT('Ctrl Pts',(-0.551949910444459,0.520737729754399,
0.0717040146871301));
#9557=CARTESIAN_POINT('Ctrl Pts',(-0.430595948725319,0.508295268527237,
0.350662848554826));
#9558=CARTESIAN_POINT('Ctrl Pts',(-0.139284333173075,0.493801248027276,
0.55472840308304));
#9559=CARTESIAN_POINT('Ctrl Pts',(0.28335615351346,0.477266726235763,0.517831802862951));
#9560=CARTESIAN_POINT('Ctrl Pts',(0.573113162045742,0.458702465869511,0.138170100375564));
#9561=CARTESIAN_POINT('Ctrl Pts',(0.487040755149608,0.44017222169388,-0.330077148654899));
#9562=CARTESIAN_POINT('Ctrl Pts',(0.0837105500021586,0.421672872730665,
-0.581703055845243));
#9563=CARTESIAN_POINT('Ctrl Pts',(-0.37380142743242,0.40320076618434,-0.45235567176097));
#9564=CARTESIAN_POINT('Ctrl Pts',(-0.561010089555589,0.386802304605621,
-0.0756527104584505));
#9565=CARTESIAN_POINT('Ctrl Pts',(-0.479552956006764,0.37246695090628,0.266522113563231));
#9566=CARTESIAN_POINT('Ctrl Pts',(-0.267488833499262,0.360187667101961,
0.478855140322724));
#9567=CARTESIAN_POINT('Ctrl Pts',(0.0742631586112486,0.34586991722832,0.559702372303342));
#9568=CARTESIAN_POINT('Ctrl Pts',(0.450399697790572,0.329517044874313,0.373843214320543));
#9569=CARTESIAN_POINT('Ctrl Pts',(0.567086603737135,0.312662109365757,-0.0443326451316622));
#9570=CARTESIAN_POINT('Ctrl Pts',(0.400224908210924,0.297344357665888,-0.383938719179592));
#9571=CARTESIAN_POINT('Ctrl Pts',(0.0660979817878402,0.282029157249401,
-0.56509208661935));
#9572=CARTESIAN_POINT('Ctrl Pts',(-0.276929936242163,0.268246205655378,
-0.48268043415828));
#9573=CARTESIAN_POINT('Ctrl Pts',(-0.493245643443692,0.254462036591453,
-0.229548648448914));
#9574=CARTESIAN_POINT('Ctrl Pts',(-0.551295150396298,0.242207808252135,
0.0671188908067961));
#9575=CARTESIAN_POINT('Ctrl Pts',(-0.40766150283296,0.228418090582837,0.377257404939042));
#9576=CARTESIAN_POINT('Ctrl Pts',(-0.110374003483933,0.214623123412753,
0.544510067179701));
#9577=CARTESIAN_POINT('Ctrl Pts',(0.229047329307677,0.200821415024854,0.506551175681503));
#9578=CARTESIAN_POINT('Ctrl Pts',(0.482289890064134,0.18701212633461,0.277245974053173));
#9579=CARTESIAN_POINT('Ctrl Pts',(0.553763732742827,0.173191747342348,-0.0573989645046387));
#9580=CARTESIAN_POINT('Ctrl Pts',(0.416146086422155,0.159363348118548,-0.370243292897184));
#9581=CARTESIAN_POINT('Ctrl Pts',(0.0882708030427006,0.143977745088325,
-0.565053420420048));
#9582=CARTESIAN_POINT('Ctrl Pts',(-0.338462248411882,0.12705070506418,-0.480836123882888));
#9583=CARTESIAN_POINT('Ctrl Pts',(-0.584075679141621,0.108515922097861,
-0.0723729196787201));
#9584=CARTESIAN_POINT('Ctrl Pts',(-0.4585052544005,0.0915751768415844,0.344428446786955));
#9585=CARTESIAN_POINT('Ctrl Pts',(-0.132406193515106,0.076005890905876,
0.5461393872929));
#9586=CARTESIAN_POINT('Ctrl Pts',(0.155419901809077,0.064566620841489,0.523143450471739));
#9587=CARTESIAN_POINT('Ctrl Pts',(0.34359217210679,0.054902908379379,0.412155588816351));
#9588=CARTESIAN_POINT('Ctrl Pts',(0.437001774418032,0.0496765590551313,
0.303330442803063));
#9589=CARTESIAN_POINT('Ctrl Pts',(0.487978555806356,0.0447398499197174,
0.206365118213754));
#9590=CARTESIAN_POINT('Ctrl Pts',(0.520046729613095,0.0393406257213133,
0.111267345674666));
#9591=CARTESIAN_POINT('Ctrl Pts',(0.533315915563189,0.0332661260171643,
-0.0318866342588667));
#9592=CARTESIAN_POINT('Ctrl Pts',(0.529475094326102,0.0345864750367511,
-0.284709647833573));
#9593=CARTESIAN_POINT('Ctrl Pts',(0.526637602108816,0.0367145593105412,
-0.544396520018928));
#9594=CARTESIAN_POINT('Ctrl Pts',(0.528538249039279,0.0353675670609071,
-0.780070492797932));
#9595=CARTESIAN_POINT('Ctrl Pts',(0.528692709166738,0.0352936010092843,
-1.10324464383216));
#9596=CARTESIAN_POINT('Ctrl Pts',(0.527761919981528,0.0359080598807752,
-1.51525401386864));
#9597=CARTESIAN_POINT('Ctrl Pts',(0.528580216238454,0.0353612811721935,
-1.83617216061816));
#9598=CARTESIAN_POINT('Ctrl Pts',(0.528325516000818,0.0355351383793534,
-1.99985072236852));
#9599=CARTESIAN_POINT('',(2.00015071794412,0.804475523135573,-0.666497406911305));
#9600=CARTESIAN_POINT('Origin',(1.99999999999998,0.759999999999999,-0.60000000000007));
#9601=CARTESIAN_POINT('',(0.662463988280159,-0.0499822726657336,-2.00015029073282));
#9602=CARTESIAN_POINT('Ctrl Pts',(2.00015071794412,0.804475523135573,-0.666497406911305));
#9603=CARTESIAN_POINT('Ctrl Pts',(1.83620821687538,0.804649660698633,-0.66675251787415));
#9604=CARTESIAN_POINT('Ctrl Pts',(1.51421119194035,0.804093904068503,-0.665928948647562));
#9605=CARTESIAN_POINT('Ctrl Pts',(1.10459263968738,0.804724235202262,-0.66687751216757));
#9606=CARTESIAN_POINT('Ctrl Pts',(0.778488091977107,0.804624888614752,-0.666703265676913));
#9607=CARTESIAN_POINT('Ctrl Pts',(0.54442707625171,0.8033242699894,-0.664844003722482));
#9608=CARTESIAN_POINT('Ctrl Pts',(0.288027302850487,0.805335668320584,-0.667586118918959));
#9609=CARTESIAN_POINT('Ctrl Pts',(0.0321180206196141,0.806907294366097,
-0.671653874643804));
#9610=CARTESIAN_POINT('Ctrl Pts',(-0.139596638836966,0.799988366367406,
-0.657366153595634));
#9611=CARTESIAN_POINT('Ctrl Pts',(-0.265956682682317,0.792781771671027,
-0.614881276898037));
#9612=CARTESIAN_POINT('Ctrl Pts',(-0.386340473147736,0.786669200591926,
-0.551372175845378));
#9613=CARTESIAN_POINT('Ctrl Pts',(-0.523816993927788,0.780063785948551,
-0.433645748061385));
#9614=CARTESIAN_POINT('Ctrl Pts',(-0.666219044663549,0.767653433960867,
-0.192704218915611));
#9615=CARTESIAN_POINT('Ctrl Pts',(-0.689058767063034,0.756222082569521,
0.0984146554749596));
#9616=CARTESIAN_POINT('Ctrl Pts',(-0.592478248153049,0.74570751472679,0.326342499792088));
#9617=CARTESIAN_POINT('Ctrl Pts',(-0.510250580429896,0.739824441432273,
0.439145396424497));
#9618=CARTESIAN_POINT('Ctrl Pts',(-0.328971586153759,0.728968689390915,
0.621190836988033));
#9619=CARTESIAN_POINT('Ctrl Pts',(0.0958337440893244,0.711671376372341,
0.74830999711301));
#9620=CARTESIAN_POINT('Ctrl Pts',(0.620304111002753,0.687911568470837,0.433769461113443));
#9621=CARTESIAN_POINT('Ctrl Pts',(0.73835387107679,0.664111160627632,-0.166965130048199));
#9622=CARTESIAN_POINT('Ctrl Pts',(0.414715655942592,0.642922729480766,-0.603621999120373));
#9623=CARTESIAN_POINT('Ctrl Pts',(-0.0275908863199736,0.62436100859898,
-0.710669286038228));
#9624=CARTESIAN_POINT('Ctrl Pts',(-0.39813025511233,0.608437064253082,-0.590670145737896));
#9625=CARTESIAN_POINT('Ctrl Pts',(-0.650080156703408,0.592499998475874,
-0.292288521076879));
#9626=CARTESIAN_POINT('Ctrl Pts',(-0.707144881750632,0.57655098007586,0.0945309854926571));
#9627=CARTESIAN_POINT('Ctrl Pts',(-0.55158365946692,0.56059094898577,0.452401551542145));
#9628=CARTESIAN_POINT('Ctrl Pts',(-0.1772094561828,0.541959207305282,0.714834645121414));
#9629=CARTESIAN_POINT('Ctrl Pts',(0.367484330759339,0.520650735211898,0.667598289986901));
#9630=CARTESIAN_POINT('Ctrl Pts',(0.742175157663465,0.496662180030771,0.177201798791322));
#9631=CARTESIAN_POINT('Ctrl Pts',(0.630965640778732,0.472660315479601,-0.429375166251397));
#9632=CARTESIAN_POINT('Ctrl Pts',(0.107586035230619,0.448648433132338,-0.756188390862319));
#9633=CARTESIAN_POINT('Ctrl Pts',(-0.487350453008389,0.424630334656425,
-0.588208599365547));
#9634=CARTESIAN_POINT('Ctrl Pts',(-0.731235197502955,0.403278517609434,
-0.0977683708505558));
#9635=CARTESIAN_POINT('Ctrl Pts',(-0.625117601034868,0.384596133557627,
0.348183842295094));
#9636=CARTESIAN_POINT('Ctrl Pts',(-0.348606790473969,0.368583951861805,
0.625079898555237));
#9637=CARTESIAN_POINT('Ctrl Pts',(0.0972167907293641,0.34990603829391,0.730574719890591));
#9638=CARTESIAN_POINT('Ctrl Pts',(0.588086029972563,0.328565375698038,0.488053495238463));
#9639=CARTESIAN_POINT('Ctrl Pts',(0.740365136709862,0.306568406437996,-0.0577085025886233));
#9640=CARTESIAN_POINT('Ctrl Pts',(0.522621279421028,0.286581789189134,-0.500819963452499));
#9641=CARTESIAN_POINT('Ctrl Pts',(0.0867941523773002,0.266605918529927,
-0.737064913155744));
#9642=CARTESIAN_POINT('Ctrl Pts',(-0.36030002070441,0.248640851668397,-0.629569645495563));
#9643=CARTESIAN_POINT('Ctrl Pts',(-0.641992299862074,0.230688881084643,
-0.299876917809462));
#9644=CARTESIAN_POINT('Ctrl Pts',(-0.717478987054585,0.214742051156983,
0.086194632105411));
#9645=CARTESIAN_POINT('Ctrl Pts',(-0.530690929834931,0.196817259725453,
0.489300976461692));
#9646=CARTESIAN_POINT('Ctrl Pts',(-0.144725676703892,0.178909769816401,
0.70633098622582));
#9647=CARTESIAN_POINT('Ctrl Pts',(0.295215046776041,0.161020056779893,0.657018975821946));
#9648=CARTESIAN_POINT('Ctrl Pts',(0.622824528841228,0.143151007884386,0.360207879087552));
#9649=CARTESIAN_POINT('Ctrl Pts',(0.715006044039375,0.125301300434412,-0.0720347673296787));
#9650=CARTESIAN_POINT('Ctrl Pts',(0.53747991286649,0.107478289621193,-0.475188997283933));
#9651=CARTESIAN_POINT('Ctrl Pts',(0.115758946274973,0.0876905285771165,
-0.725599039992233));
#9652=CARTESIAN_POINT('Ctrl Pts',(-0.431538112822807,0.0659892634348224,
-0.617104732797172));
#9653=CARTESIAN_POINT('Ctrl Pts',(-0.744693743478759,0.0422927786570434,
-0.0951523515529584));
#9654=CARTESIAN_POINT('Ctrl Pts',(-0.585085784735021,0.0207569079373872,
0.435755076168825));
#9655=CARTESIAN_POINT('Ctrl Pts',(-0.170310845287768,0.00096264921625724,
0.690490277729099));
#9656=CARTESIAN_POINT('Ctrl Pts',(0.191480329024041,-0.0134075415523006,
0.662765347245377));
#9657=CARTESIAN_POINT('Ctrl Pts',(0.431002395435098,-0.0256993836631372,
0.520971575878654));
#9658=CARTESIAN_POINT('Ctrl Pts',(0.548065973192159,-0.032280894159065,
0.384307758714896));
#9659=CARTESIAN_POINT('Ctrl Pts',(0.611163697009464,-0.0383525034286994,
0.264648815779984));
#9660=CARTESIAN_POINT('Ctrl Pts',(0.65335380658105,-0.0455068140358546,
0.139218056313768));
#9661=CARTESIAN_POINT('Ctrl Pts',(0.667640080240138,-0.0524139639419364,
-0.0320317672708526));
#9662=CARTESIAN_POINT('Ctrl Pts',(0.663563470597623,-0.0508446374556383,
-0.288026483088336));
#9663=CARTESIAN_POINT('Ctrl Pts',(0.660820022877162,-0.0488315955858374,
-0.544415125004604));
#9664=CARTESIAN_POINT('Ctrl Pts',(0.662676266642772,-0.050132523365314,
-0.778488486630415));
#9665=CARTESIAN_POINT('Ctrl Pts',(0.662849183916153,-0.050231417425612,
-1.10458538375921));
#9666=CARTESIAN_POINT('Ctrl Pts',(0.661897332210143,-0.0496009500256405,
-1.51421284590545));
#9667=CARTESIAN_POINT('Ctrl Pts',(0.662719098649113,-0.050156409826639,
-1.8362081654112));
#9668=CARTESIAN_POINT('Ctrl Pts',(0.662463988280159,-0.0499822726657336,
-2.00015029073282));
#9669=CARTESIAN_POINT('Origin',(0.6,0.,-2.));
#9670=CARTESIAN_POINT('Ctrl Pts',(0.600124355483126,-0.0799998580128369,
-2.00008516830249));
#9671=CARTESIAN_POINT('Ctrl Pts',(0.600379376695518,-0.0801739343158842,
-1.83620033785433));
#9672=CARTESIAN_POINT('Ctrl Pts',(0.599562611053881,-0.0796184124528264,
-1.5144754520526));
#9673=CARTESIAN_POINT('Ctrl Pts',(0.600502518404447,-0.0802525034314073,
-1.10424411057565));
#9674=CARTESIAN_POINT('Ctrl Pts',(0.600344602427935,-0.0801506833161176,
-0.778901942331774));
#9675=CARTESIAN_POINT('Ctrl Pts',(0.598456953704134,-0.0788587712934794,
-0.544242160533997));
#9676=CARTESIAN_POINT('Ctrl Pts',(0.601272474507003,-0.0808543685860998,
-0.287680267082095));
#9677=CARTESIAN_POINT('Ctrl Pts',(0.605184477979747,-0.0824681761820383,
-0.0307556431383126));
#9678=CARTESIAN_POINT('Ctrl Pts',(0.588609512632607,-0.0742202560328195,
0.161001223625551));
#9679=CARTESIAN_POINT('Ctrl Pts',(0.518063450209372,-0.0648906358873938,
0.323627369018429));
#9680=CARTESIAN_POINT('Ctrl Pts',(0.389740128736442,-0.0579722786893707,
0.474748184678881));
#9681=CARTESIAN_POINT('Ctrl Pts',(0.173020606908044,-0.0467144436845919,
0.602178110487582));
#9682=CARTESIAN_POINT('Ctrl Pts',(-0.156647509262585,-0.0336993466160229,
0.628366170043479));
#9683=CARTESIAN_POINT('Ctrl Pts',(-0.534302969503257,-0.01563383198389,
0.396152535345114));
#9684=CARTESIAN_POINT('Ctrl Pts',(-0.680181221263981,0.00400588873282267,
-0.0887030397692518));
#9685=CARTESIAN_POINT('Ctrl Pts',(-0.465603142330848,0.0202821362637637,
-0.446134214125788));
#9686=CARTESIAN_POINT('Ctrl Pts',(-0.165486932860075,0.03474270768116,-0.612245575240685));
#9687=CARTESIAN_POINT('Ctrl Pts',(0.146295095787791,0.0474352484480225,
-0.642641412885972));
#9688=CARTESIAN_POINT('Ctrl Pts',(0.495949774692522,0.0637997238881112,
-0.436123139243827));
#9689=CARTESIAN_POINT('Ctrl Pts',(0.659385538859151,0.0802233041204479,
-0.0644782106763051));
#9690=CARTESIAN_POINT('Ctrl Pts',(0.574545201045043,0.0966991572901908,
0.334449484668907));
#9691=CARTESIAN_POINT('Ctrl Pts',(0.271532605139402,0.113229721085999,0.609171048717871));
#9692=CARTESIAN_POINT('Ctrl Pts',(-0.136251969463658,0.129813195665052,
0.654997123118035));
#9693=CARTESIAN_POINT('Ctrl Pts',(-0.494901592911036,0.146449576154649,
0.453502429895765));
#9694=CARTESIAN_POINT('Ctrl Pts',(-0.668917284177339,0.163138203343486,
0.0782620703516101));
#9695=CARTESIAN_POINT('Ctrl Pts',(-0.598644996586867,0.178018517289954,
-0.282046799603755));
#9696=CARTESIAN_POINT('Ctrl Pts',(-0.335262243900907,0.194801447000121,
-0.590258574308657));
#9697=CARTESIAN_POINT('Ctrl Pts',(0.0833281156314849,0.211635077569448,
-0.691395156339746));
#9698=CARTESIAN_POINT('Ctrl Pts',(0.4320119853653,0.227588446215705,-0.502587368796631));
#9699=CARTESIAN_POINT('Ctrl Pts',(0.58527223262087,0.238874211068699,-0.281979562605746));
#9700=CARTESIAN_POINT('Ctrl Pts',(0.678917739338141,0.252059849462334,0.0184388692246381));
#9701=CARTESIAN_POINT('Ctrl Pts',(0.554821413577227,0.270001502682695,0.463024783480917));
#9702=CARTESIAN_POINT('Ctrl Pts',(0.089888824047859,0.290221470828933,0.693551038003489));
#9703=CARTESIAN_POINT('Ctrl Pts',(-0.272915151999609,0.305432097922516,
0.607393400489082));
#9704=CARTESIAN_POINT('Ctrl Pts',(-0.465626168527264,0.315590515005467,
0.46173311346713));
#9705=CARTESIAN_POINT('Ctrl Pts',(-0.611423927492396,0.325760833794014,
0.268821318511434));
#9706=CARTESIAN_POINT('Ctrl Pts',(-0.698650473779508,0.341042831595186,
-0.0956472554953462));
#9707=CARTESIAN_POINT('Ctrl Pts',(-0.465321982498693,0.361476665326508,
-0.565350807747607));
#9708=CARTESIAN_POINT('Ctrl Pts',(0.10575120321005,0.38454069790763,-0.726974188805798));
#9709=CARTESIAN_POINT('Ctrl Pts',(0.610387251745808,0.407678360873112,-0.412408779209339));
#9710=CARTESIAN_POINT('Ctrl Pts',(0.718323895495084,0.430887045922702,0.17413060542287));
#9711=CARTESIAN_POINT('Ctrl Pts',(0.355237119019683,0.454164351458316,0.650683811024646));
#9712=CARTESIAN_POINT('Ctrl Pts',(-0.175382406590221,0.4749142230429,0.695878649309196));
#9713=CARTESIAN_POINT('Ctrl Pts',(-0.54101475967607,0.49311138275633,0.440269492223299));
#9714=CARTESIAN_POINT('Ctrl Pts',(-0.693527526572458,0.50873629806685,0.0898379898580044));
#9715=CARTESIAN_POINT('Ctrl Pts',(-0.646735970560938,0.521779183073869,
-0.226461651899009));
#9716=CARTESIAN_POINT('Ctrl Pts',(-0.513906112786406,0.532226370805735,
-0.436433419735239));
#9717=CARTESIAN_POINT('Ctrl Pts',(-0.328920782360512,0.542681936352062,
-0.602852159734885));
#9718=CARTESIAN_POINT('Ctrl Pts',(-0.0243494995865983,0.55576702001899,
-0.701905622444322));
#9719=CARTESIAN_POINT('Ctrl Pts',(0.318684360355662,0.570182439320145,-0.618057422392217));
#9720=CARTESIAN_POINT('Ctrl Pts',(0.554275268889935,0.583304705413154,-0.407908493988256));
#9721=CARTESIAN_POINT('Ctrl Pts',(0.713586310862138,0.599067032359038,-0.0629718800249659));
#9722=CARTESIAN_POINT('Ctrl Pts',(0.617323759198901,0.61880473745743,0.433855029903579));
#9723=CARTESIAN_POINT('Ctrl Pts',(0.0931818027763926,0.642526983889894,
0.749181117386836));
#9724=CARTESIAN_POINT('Ctrl Pts',(-0.314313763037281,0.659133011706964,
0.627311226200405));
#9725=CARTESIAN_POINT('Ctrl Pts',(-0.477269723836412,0.668539639010893,
0.476341934975343));
#9726=CARTESIAN_POINT('Ctrl Pts',(-0.524957853949116,0.671513213020625,
0.424882768662061));
#9727=CARTESIAN_POINT('Ctrl Pts',(-0.597179322807005,0.676677358782867,
0.325569816011966));
#9728=CARTESIAN_POINT('Ctrl Pts',(-0.69448376569806,0.6873032670482,0.0964041117283874));
#9729=CARTESIAN_POINT('Ctrl Pts',(-0.671478747098358,0.69869719950028,-0.197322255866813));
#9730=CARTESIAN_POINT('Ctrl Pts',(-0.527686488423399,0.711441182605667,
-0.440569074748579));
#9731=CARTESIAN_POINT('Ctrl Pts',(-0.36114955668007,0.719020822056164,-0.583433135906584));
#9732=CARTESIAN_POINT('Ctrl Pts',(-0.171544666302877,0.729888896055897,
-0.664752607658936));
#9733=CARTESIAN_POINT('Ctrl Pts',(0.0327819626725445,0.738541246775484,
-0.681326463162123));
#9734=CARTESIAN_POINT('Ctrl Pts',(0.287281763425397,0.736796378226309,-0.677467579294977));
#9735=CARTESIAN_POINT('Ctrl Pts',(0.544477498698488,0.734860197456536,-0.674632411152923));
#9736=CARTESIAN_POINT('Ctrl Pts',(0.778765801010588,0.736127346477361,-0.676530344298986));
#9737=CARTESIAN_POINT('Ctrl Pts',(1.10435275137728,0.736241519844584,-0.676684603908725));
#9738=CARTESIAN_POINT('Ctrl Pts',(1.51439530422594,0.735599108498541,-0.675749139626198));
#9739=CARTESIAN_POINT('Ctrl Pts',(1.83620130898864,0.736158775205915,-0.676565295388702));
#9740=CARTESIAN_POINT('Ctrl Pts',(2.00009323767342,0.735984691360175,-0.676310263121555));
#9741=CARTESIAN_POINT('Ctrl Pts',(0.623974753147584,-0.0799627443810934,
-2.00012224248872));
#9742=CARTESIAN_POINT('Ctrl Pts',(0.624229825439503,-0.0801368555507905,
-1.83620458669381));
#9743=CARTESIAN_POINT('Ctrl Pts',(0.623412063162941,-0.0795796261306918,
-1.51433796979021));
#9744=CARTESIAN_POINT('Ctrl Pts',(0.624359859480197,-0.0802179503669397,
-1.10443039061536));
#9745=CARTESIAN_POINT('Ctrl Pts',(0.62419562566126,-0.0801105878584707,
-0.778694387346514));
#9746=CARTESIAN_POINT('Ctrl Pts',(0.622325145889363,-0.0788301395864106,
-0.544301413101009));
#9747=CARTESIAN_POINT('Ctrl Pts',(0.625106583269737,-0.0807989774146498,
-0.288007276047959));
#9748=CARTESIAN_POINT('Ctrl Pts',(0.629104794486704,-0.0824730503396987,
-0.031111740534322));
#9749=CARTESIAN_POINT('Ctrl Pts',(0.612250467993575,-0.0740274841813297,
0.166374233370359));
#9750=CARTESIAN_POINT('Ctrl Pts',(0.538550980620464,-0.0642460178139413,
0.336780746391469));
#9751=CARTESIAN_POINT('Ctrl Pts',(0.405452154198712,-0.057098070267831,
0.493123831974176));
#9752=CARTESIAN_POINT('Ctrl Pts',(0.179790463925493,-0.045362414675718,
0.626129196125436));
#9753=CARTESIAN_POINT('Ctrl Pts',(-0.162515835153933,-0.0318610350483913,
0.652948899440053));
#9754=CARTESIAN_POINT('Ctrl Pts',(-0.555104121078402,-0.013076772153776,
0.411861924804563));
#9755=CARTESIAN_POINT('Ctrl Pts',(-0.706494995716607,0.00731586852288217,
-0.0919341536269851));
#9756=CARTESIAN_POINT('Ctrl Pts',(-0.483689317242129,0.0242199786601462,
-0.463046839212734));
#9757=CARTESIAN_POINT('Ctrl Pts',(-0.172085161128402,0.0392327419485987,
-0.635510782103407));
#9758=CARTESIAN_POINT('Ctrl Pts',(0.151534851775174,0.0524067893783082,
-0.667051829582526));
#9759=CARTESIAN_POINT('Ctrl Pts',(0.514342017305476,0.0693857790668076,
-0.452740521293047));
#9760=CARTESIAN_POINT('Ctrl Pts',(0.68385146227568,0.0864208989509592,-0.0672288061262263));
#9761=CARTESIAN_POINT('Ctrl Pts',(0.595856693475746,0.103503527696193,0.346416299319125));
#9762=CARTESIAN_POINT('Ctrl Pts',(0.281766337021811,0.120636343208791,0.631146960462356));
#9763=CARTESIAN_POINT('Ctrl Pts',(-0.140730452143404,0.137816821820559,
0.67859963752343));
#9764=CARTESIAN_POINT('Ctrl Pts',(-0.512143481669323,0.15504448338329,0.469904875349947));
#9765=CARTESIAN_POINT('Ctrl Pts',(-0.692248298424958,0.172318474499937,
0.0814608902124625));
#9766=CARTESIAN_POINT('Ctrl Pts',(-0.619518631402499,0.187712934444724,
-0.291320794134974));
#9767=CARTESIAN_POINT('Ctrl Pts',(-0.347101977382683,0.205069580874819,
-0.610083796980475));
#9768=CARTESIAN_POINT('Ctrl Pts',(0.0856264740795014,0.222470485013252,
-0.714571021120727));
#9769=CARTESIAN_POINT('Ctrl Pts',(0.44580046722091,0.238948816751437,-0.519495022345486));
#9770=CARTESIAN_POINT('Ctrl Pts',(0.604066108994964,0.25060297477869,-0.291675312775178));
#9771=CARTESIAN_POINT('Ctrl Pts',(0.700738910463294,0.264215420555072,0.0184849426418081));
#9772=CARTESIAN_POINT('Ctrl Pts',(0.572640898984596,0.282723178790392,0.477162825367339));
#9773=CARTESIAN_POINT('Ctrl Pts',(0.0932568014054071,0.303568974758758,
0.714756971115007));
#9774=CARTESIAN_POINT('Ctrl Pts',(-0.280540254320519,0.319240073683042,
0.625960485616185));
#9775=CARTESIAN_POINT('Ctrl Pts',(-0.479004310712579,0.32970135829011,0.47594246027192));
#9776=CARTESIAN_POINT('Ctrl Pts',(-0.629123425868339,0.340173193562948,
0.277305322213801));
#9777=CARTESIAN_POINT('Ctrl Pts',(-0.718857967185726,0.355898871371537,
-0.0977904793576591));
#9778=CARTESIAN_POINT('Ctrl Pts',(-0.478821925431186,0.376910052425976,
-0.580774275577745));
#9779=CARTESIAN_POINT('Ctrl Pts',(0.107973512819069,0.40060519253458,-0.746719455522737));
#9780=CARTESIAN_POINT('Ctrl Pts',(0.625924802892503,0.424354169765414,-0.423710203648399));
#9781=CARTESIAN_POINT('Ctrl Pts',(0.736504811271342,0.448152928948129,0.177837918946914));
#9782=CARTESIAN_POINT('Ctrl Pts',(0.36440052610237,0.471999615636857,0.666006076478248));
#9783=CARTESIAN_POINT('Ctrl Pts',(-0.178677986430279,0.493233270995688,
0.712167492060102));
#9784=CARTESIAN_POINT('Ctrl Pts',(-0.552580736158049,0.511842586077471,
0.450719359413262));
#9785=CARTESIAN_POINT('Ctrl Pts',(-0.708421284622368,0.527810293363266,
0.0925696490070121));
#9786=CARTESIAN_POINT('Ctrl Pts',(-0.660610117307273,0.541126816837653,
-0.230412043824339));
#9787=CARTESIAN_POINT('Ctrl Pts',(-0.525019612582926,0.551790527195324,
-0.444737715779806));
#9788=CARTESIAN_POINT('Ctrl Pts',(-0.336266792259839,0.562457991275901,
-0.6145419193976));
#9789=CARTESIAN_POINT('Ctrl Pts',(-0.0256559250583661,0.575801054431563,
-0.715518174515178));
#9790=CARTESIAN_POINT('Ctrl Pts',(0.323914068012285,0.590490635965341,-0.630042052906425));
#9791=CARTESIAN_POINT('Ctrl Pts',(0.563820115939216,0.603852583815099,-0.416011490533624));
#9792=CARTESIAN_POINT('Ctrl Pts',(0.725951907577493,0.619896011193044,-0.0648918311942802));
#9793=CARTESIAN_POINT('Ctrl Pts',(0.627947962839659,0.639966556187965,0.440373284353448));
#9794=CARTESIAN_POINT('Ctrl Pts',(0.0954058193471724,0.664062078710943,
0.760535410298491));
#9795=CARTESIAN_POINT('Ctrl Pts',(-0.317995504911745,0.680907415525936,
0.636799082423208));
#9796=CARTESIAN_POINT('Ctrl Pts',(-0.483264921611616,0.690447266925411,
0.483685722801391));
#9797=CARTESIAN_POINT('Ctrl Pts',(-0.531624460286487,0.693462936034065,
0.43149728805094));
#9798=CARTESIAN_POINT('Ctrl Pts',(-0.604845284247209,0.698696869474255,
0.330839773996165));
#9799=CARTESIAN_POINT('Ctrl Pts',(-0.703408711992183,0.709469969798145,
0.0984987021510025));
#9800=CARTESIAN_POINT('Ctrl Pts',(-0.680229358189844,0.720995021434779,
-0.198734448803209));
#9801=CARTESIAN_POINT('Ctrl Pts',(-0.534484562592715,0.733907467506484,
-0.445150691856127));
#9802=CARTESIAN_POINT('Ctrl Pts',(-0.366079777526243,0.74156757604019,-0.589608759958203));
#9803=CARTESIAN_POINT('Ctrl Pts',(-0.174590108750424,0.752554221350636,
-0.671730400299516));
#9804=CARTESIAN_POINT('Ctrl Pts',(0.0327210575797316,0.761314607562119,
-0.688577883529026));
#9805=CARTESIAN_POINT('Ctrl Pts',(0.287711988942633,0.759538617285864,-0.684617964692094));
#9806=CARTESIAN_POINT('Ctrl Pts',(0.544497969015785,0.757615772552647,-0.681818632137197));
#9807=CARTESIAN_POINT('Ctrl Pts',(0.778596989996061,0.758876900759646,-0.683695542906545));
#9808=CARTESIAN_POINT('Ctrl Pts',(1.10452217702354,0.75899378202524,-0.683855618983067));
#9809=CARTESIAN_POINT('Ctrl Pts',(1.51427783815987,0.758348873032374,-0.682909105628775));
#9810=CARTESIAN_POINT('Ctrl Pts',(1.83620533625635,0.758909242853562,-0.683725002411278));
#9811=CARTESIAN_POINT('Ctrl Pts',(2.00012854403087,0.758735125783585,-0.683469921470732));
#9812=CARTESIAN_POINT('Ctrl Pts',(0.647562717600109,-0.0686047413844538,
-2.00014688340338));
#9813=CARTESIAN_POINT('Ctrl Pts',(0.647817823654385,-0.06877887560018,-1.8362075308324));
#9814=CARTESIAN_POINT('Ctrl Pts',(0.646999311251896,-0.0682200876930409,
-1.51424075188625));
#9815=CARTESIAN_POINT('Ctrl Pts',(0.647951340387484,-0.0688620337896085,
-1.1045587808546));
#9816=CARTESIAN_POINT('Ctrl Pts',(0.647783322613642,-0.0687497485883994,
-0.778544160373208));
#9817=CARTESIAN_POINT('Ctrl Pts',(0.645922404729212,-0.0674793762396106,
-0.544360858002009));
#9818=CARTESIAN_POINT('Ctrl Pts',(0.648684014072772,-0.0694244873789363,
-0.288166569069797));
#9819=CARTESIAN_POINT('Ctrl Pts',(0.652730727559635,-0.0711516627382978,
-0.0315529265726239));
#9820=CARTESIAN_POINT('Ctrl Pts',(0.635698168786289,-0.0625351806976687,
0.170966473990833));
#9821=CARTESIAN_POINT('Ctrl Pts',(0.558803449129216,-0.0522976255106795,
0.349303642561896));
#9822=CARTESIAN_POINT('Ctrl Pts',(0.421064255675426,-0.044928704997045,
0.510662776778674));
#9823=CARTESIAN_POINT('Ctrl Pts',(0.186782551168435,-0.0327314990430446,
0.649051524597898));
#9824=CARTESIAN_POINT('Ctrl Pts',(-0.167675538339671,-0.0187626080188767,
0.67645878212063));
#9825=CARTESIAN_POINT('Ctrl Pts',(-0.574346007811733,0.000701651077454804,
0.426944282706536));
#9826=CARTESIAN_POINT('Ctrl Pts',(-0.730818163437985,0.021796163491512,
-0.0945071158682554));
#9827=CARTESIAN_POINT('Ctrl Pts',(-0.500435617268145,0.0392746662117698,
-0.478086738213446));
#9828=CARTESIAN_POINT('Ctrl Pts',(-0.178473613097707,0.0547855760479349,
-0.656278999259023));
#9829=CARTESIAN_POINT('Ctrl Pts',(0.155739197633759,0.0683907912820399,
-0.688814955739565));
#9830=CARTESIAN_POINT('Ctrl Pts',(0.530114084533772,0.0859119083272224,
-0.467609708028388));
#9831=CARTESIAN_POINT('Ctrl Pts',(0.704861976973911,0.10347820932996,-0.0700557074029037));
#9832=CARTESIAN_POINT('Ctrl Pts',(0.614140928007568,0.121079751027447,0.356150243253928));
#9833=CARTESIAN_POINT('Ctrl Pts',(0.290720381570364,0.138719347207698,0.649264750912455));
#9834=CARTESIAN_POINT('Ctrl Pts',(-0.143935197576834,0.156393884255417,
0.698027557862093));
#9835=CARTESIAN_POINT('Ctrl Pts',(-0.525695989392685,0.174102555769698,
0.483454429524658));
#9836=CARTESIAN_POINT('Ctrl Pts',(-0.71062298823528,0.191844238327655,0.0844656496154849));
#9837=CARTESIAN_POINT('Ctrl Pts',(-0.635941273898295,0.207642191616313,
-0.298078404553257));
#9838=CARTESIAN_POINT('Ctrl Pts',(-0.35655077793279,0.225441229907459,-0.624951269652307));
#9839=CARTESIAN_POINT('Ctrl Pts',(0.0868534510073472,0.243270380020131,
-0.73191354407885));
#9840=CARTESIAN_POINT('Ctrl Pts',(0.455477411176392,0.260136813586793,-0.532183195716537));
#9841=CARTESIAN_POINT('Ctrl Pts',(0.617357217331075,0.27205767557878,-0.299148538315059));
#9842=CARTESIAN_POINT('Ctrl Pts',(0.71618836382869,0.285975427384868,0.0179807600873472));
#9843=CARTESIAN_POINT('Ctrl Pts',(0.585204956240556,0.304882369925317,0.486524353131866));
#9844=CARTESIAN_POINT('Ctrl Pts',(0.0960129954608337,0.326152254444956,
0.728829046239284));
#9845=CARTESIAN_POINT('Ctrl Pts',(-0.284982589881197,0.342125765179505,
0.638272956156149));
#9846=CARTESIAN_POINT('Ctrl Pts',(-0.487146226499544,0.352782283843396,
0.485449782328244));
#9847=CARTESIAN_POINT('Ctrl Pts',(-0.639999877979491,0.363445193023275,
0.283183469426195));
#9848=CARTESIAN_POINT('Ctrl Pts',(-0.731267396964867,0.379447632097204,
-0.0985338428943742));
#9849=CARTESIAN_POINT('Ctrl Pts',(-0.487133911852248,0.400806088810658,
-0.589443413007349));
#9850=CARTESIAN_POINT('Ctrl Pts',(0.108652013139086,0.424862211386592,-0.757752991265812));
#9851=CARTESIAN_POINT('Ctrl Pts',(0.633727981828975,0.448941962928639,-0.430101733974972));
#9852=CARTESIAN_POINT('Ctrl Pts',(0.74553666345861,0.473040826939442,0.179067888189971));
#9853=CARTESIAN_POINT('Ctrl Pts',(0.369092302572918,0.497156637125847,0.672639049653024));
#9854=CARTESIAN_POINT('Ctrl Pts',(-0.179399554126267,0.518601582525948,
0.719112270123592));
#9855=CARTESIAN_POINT('Ctrl Pts',(-0.556567621013042,0.537375388258511,
0.455307243010448));
#9856=CARTESIAN_POINT('Ctrl Pts',(-0.713604967963102,0.553469940848612,
0.0942917727417075));
#9857=CARTESIAN_POINT('Ctrl Pts',(-0.665414559125122,0.566880235417034,
-0.230958493782574));
#9858=CARTESIAN_POINT('Ctrl Pts',(-0.528954541427128,0.57761190439304,-0.446644246401335));
#9859=CARTESIAN_POINT('Ctrl Pts',(-0.339076478980064,0.588342534616196,
-0.617449336631183));
#9860=CARTESIAN_POINT('Ctrl Pts',(-0.0268235233283263,0.601755594253088,
-0.718916870502273));
#9861=CARTESIAN_POINT('Ctrl Pts',(0.324255474853437,0.616509012230526,-0.633024580536174));
#9862=CARTESIAN_POINT('Ctrl Pts',(0.56499789305728,0.629918454098719,-0.41821910925962));
#9863=CARTESIAN_POINT('Ctrl Pts',(0.727572156699319,0.646008086207112,-0.0660687241023528));
#9864=CARTESIAN_POINT('Ctrl Pts',(0.629246955383781,0.666115997057895,0.440121077839912));
#9865=CARTESIAN_POINT('Ctrl Pts',(0.0963360596202998,0.690223883850523,
0.760285666107944));
#9866=CARTESIAN_POINT('Ctrl Pts',(-0.316678988048333,0.707054904105865,
0.63654207486579));
#9867=CARTESIAN_POINT('Ctrl Pts',(-0.481687401461808,0.716579782808358,
0.483670161998668));
#9868=CARTESIAN_POINT('Ctrl Pts',(-0.529964766765977,0.719590322805737,
0.431569437455635));
#9869=CARTESIAN_POINT('Ctrl Pts',(-0.603043166083147,0.724814190701037,
0.331109063559711));
#9870=CARTESIAN_POINT('Ctrl Pts',(-0.701377603074042,0.735562736341102,
0.0992698806470131));
#9871=CARTESIAN_POINT('Ctrl Pts',(-0.678208718803284,0.747052970111286,
-0.197007108721183));
#9872=CARTESIAN_POINT('Ctrl Pts',(-0.533049782551756,0.759915124360583,
-0.442527004349377));
#9873=CARTESIAN_POINT('Ctrl Pts',(-0.365130150057323,0.767553352808611,
-0.586422650312711));
#9874=CARTESIAN_POINT('Ctrl Pts',(-0.175401583891143,0.778448000940243,
-0.667878786877269));
#9875=CARTESIAN_POINT('Ctrl Pts',(0.0324402657906996,0.78723317066499,-0.684909823724877));
#9876=CARTESIAN_POINT('Ctrl Pts',(0.288015320783504,0.785452363342735,-0.680884264968639));
#9877=CARTESIAN_POINT('Ctrl Pts',(0.544474856630133,0.783531757833144,-0.678113913170131));
#9878=CARTESIAN_POINT('Ctrl Pts',(0.778496518105208,0.784792023974274,-0.679978689304889));
#9879=CARTESIAN_POINT('Ctrl Pts',(1.10461251107124,0.784909435358377,-0.680144875308017));
#9880=CARTESIAN_POINT('Ctrl Pts',(1.51420958961188,0.784264160485163,-0.679194142967422));
#9881=CARTESIAN_POINT('Ctrl Pts',(1.83620793448134,0.784824707877476,-0.680012060334172));
#9882=CARTESIAN_POINT('Ctrl Pts',(2.00015029331814,0.784650570465493,-0.679756949592654));
#9883=CARTESIAN_POINT('Ctrl Pts',(0.662463988280159,-0.0499822726657336,
-2.00015029073282));
#9884=CARTESIAN_POINT('Ctrl Pts',(0.662719098649113,-0.050156409826639,
-1.8362081654112));
#9885=CARTESIAN_POINT('Ctrl Pts',(0.661899454328382,-0.0495966927590349,
-1.51421755028528));
#9886=CARTESIAN_POINT('Ctrl Pts',(0.66284910632835,-0.0502402207575894,
-1.10458006510705));
#9887=CARTESIAN_POINT('Ctrl Pts',(0.662680367156758,-0.0501253275132676,
-0.778501033524502));
#9888=CARTESIAN_POINT('Ctrl Pts',(0.660816894629293,-0.0488599276476446,
-0.544393513999504));
#9889=CARTESIAN_POINT('Ctrl Pts',(0.663578472032617,-0.0507927293188021,
-0.288093216071113));
#9890=CARTESIAN_POINT('Ctrl Pts',(0.667616321865346,-0.05254656640794,-0.0319099260796923));
#9891=CARTESIAN_POINT('Ctrl Pts',(0.650567348477531,-0.043847011278566,
0.173143128512355));
#9892=CARTESIAN_POINT('Ctrl Pts',(0.571579298183145,-0.0333126323934734,
0.356716710686719));
#9893=CARTESIAN_POINT('Ctrl Pts',(0.430996119168082,-0.0258103364145119,
0.521087714337906));
#9894=CARTESIAN_POINT('Ctrl Pts',(0.1915071815102,-0.0133332387943894,0.662736701654699));
#9895=CARTESIAN_POINT('Ctrl Pts',(-0.170274276907979,0.000917860101533585,
0.690477633323126));
#9896=CARTESIAN_POINT('Ctrl Pts',(-0.585129454859053,0.0207803290775139,
0.435999532244355));
#9897=CARTESIAN_POINT('Ctrl Pts',(-0.744443896456613,0.0422755776723358,
-0.095507074164448));
#9898=CARTESIAN_POINT('Ctrl Pts',(-0.509841682105653,0.0600698652129145,
-0.48587284842243));
#9899=CARTESIAN_POINT('Ctrl Pts',(-0.182371420410715,0.0758462955406901,
-0.667116998551829));
#9900=CARTESIAN_POINT('Ctrl Pts',(0.157399036884807,0.0896784376807901,
-0.70013721155414));
#9901=CARTESIAN_POINT('Ctrl Pts',(0.537616507612329,0.107475858373865,-0.475407626319063));
#9902=CARTESIAN_POINT('Ctrl Pts',(0.714892343577423,0.125303248323797,-0.0719474598634416));
#9903=CARTESIAN_POINT('Ctrl Pts',(0.622850446151327,0.143150556790639,0.360164498039423));
#9904=CARTESIAN_POINT('Ctrl Pts',(0.29518893985529,0.161020474047202,0.657035729572063));
#9905=CARTESIAN_POINT('Ctrl Pts',(-0.144717629684642,0.178909688014726,
0.706323488235444));
#9906=CARTESIAN_POINT('Ctrl Pts',(-0.530705045249643,0.196817350568182,
0.489298555050095));
#9907=CARTESIAN_POINT('Ctrl Pts',(-0.717460687670318,0.214742034949024,
0.0862002289659455));
#9908=CARTESIAN_POINT('Ctrl Pts',(-0.642031232999526,0.230688899152405,
-0.29990296920214));
#9909=CARTESIAN_POINT('Ctrl Pts',(-0.360225222270616,0.248640848207253,
-0.629537751434071));
#9910=CARTESIAN_POINT('Ctrl Pts',(0.0865652378839908,0.266605936263461,
-0.737214564320495));
#9911=CARTESIAN_POINT('Ctrl Pts',(0.457579401162888,0.283585396119934,-0.536108564143753));
#9912=CARTESIAN_POINT('Ctrl Pts',(0.620386129590537,0.295575769676806,-0.301726429359565));
#9913=CARTESIAN_POINT('Ctrl Pts',(0.719733178313584,0.309567943995265,0.017099356343888));
#9914=CARTESIAN_POINT('Ctrl Pts',(0.588010276659275,0.328565400057628,0.487758585805817));
#9915=CARTESIAN_POINT('Ctrl Pts',(0.0971670852606046,0.349906037582471,
0.730730476660701));
#9916=CARTESIAN_POINT('Ctrl Pts',(-0.284652563504559,0.365915702155902,
0.639924193300074));
#9917=CARTESIAN_POINT('Ctrl Pts',(-0.487137810765924,0.376590035291017,
0.486854053066531));
#9918=CARTESIAN_POINT('Ctrl Pts',(-0.640157655994926,0.387265017474822,
0.284357621330306));
#9919=CARTESIAN_POINT('Ctrl Pts',(-0.731435491885652,0.40327851439673,-0.0976053795959151));
#9920=CARTESIAN_POINT('Ctrl Pts',(-0.487282112219958,0.424630326141765,
-0.588251513730542));
#9921=CARTESIAN_POINT('Ctrl Pts',(0.107542304304109,0.448648432219031,-0.756123031572738));
#9922=CARTESIAN_POINT('Ctrl Pts',(0.631001759798563,0.472660308219991,-0.429295319219671));
#9923=CARTESIAN_POINT('Ctrl Pts',(0.74218478195565,0.496662177151635,0.177378805470387));
#9924=CARTESIAN_POINT('Ctrl Pts',(0.367633182807851,0.520650711771743,0.668206905588921));
#9925=CARTESIAN_POINT('Ctrl Pts',(-0.177290589757161,0.541959211942665,
0.714225571639092));
#9926=CARTESIAN_POINT('Ctrl Pts',(-0.551548311632649,0.560590950253618,
0.452391321581651));
#9927=CARTESIAN_POINT('Ctrl Pts',(-0.707222318657316,0.576550987095786,
0.0943897454653029));
#9928=CARTESIAN_POINT('Ctrl Pts',(-0.659429314778723,0.589841843320291,
-0.227905593604475));
#9929=CARTESIAN_POINT('Ctrl Pts',(-0.524302856027198,0.600468553416982,
-0.441469891084629));
#9930=CARTESIAN_POINT('Ctrl Pts',(-0.336344999478411,0.611091037993889,
-0.610532913980466));
#9931=CARTESIAN_POINT('Ctrl Pts',(-0.027435641532116,0.62436110450958,-0.710885116678141));
#9932=CARTESIAN_POINT('Ctrl Pts',(0.319584613456734,0.638945190751432,-0.625937595350502));
#9933=CARTESIAN_POINT('Ctrl Pts',(0.557385963976335,0.652193001743414,-0.413741983631198));
#9934=CARTESIAN_POINT('Ctrl Pts',(0.717866358113644,0.668077414553885,-0.0660827982863029));
#9935=CARTESIAN_POINT('Ctrl Pts',(0.620756152430939,0.687913874031373,0.433187274501453));
#9936=CARTESIAN_POINT('Ctrl Pts',(0.095640770400992,0.711668836897727,0.74852107598595));
#9937=CARTESIAN_POINT('Ctrl Pts',(-0.310834112497513,0.72823701458646,0.626633342288499));
#9938=CARTESIAN_POINT('Ctrl Pts',(-0.473100780452007,0.737604098016007,
0.476301824795464));
#9939=CARTESIAN_POINT('Ctrl Pts',(-0.520571911912829,0.740564126634636,
0.42507429163648));
#9940=CARTESIAN_POINT('Ctrl Pts',(-0.592417282988213,0.745701681582158,
0.326282155767353));
#9941=CARTESIAN_POINT('Ctrl Pts',(-0.689117006009886,0.756262723952014,
0.0984423004980192));
#9942=CARTESIAN_POINT('Ctrl Pts',(-0.666140421673785,0.76756456855443,-0.192756292142937));
#9943=CARTESIAN_POINT('Ctrl Pts',(-0.523895647667715,0.780175707607948,
-0.433635461326377));
#9944=CARTESIAN_POINT('Ctrl Pts',(-0.358640415083758,0.787697519295988,
-0.575013532729149));
#9945=CARTESIAN_POINT('Ctrl Pts',(-0.173686618063833,0.798322615376446,
-0.654575062224357));
#9946=CARTESIAN_POINT('Ctrl Pts',(0.0320410938202948,0.807040382619809,
-0.671633206639044));
#9947=CARTESIAN_POINT('Ctrl Pts',(0.288083260014899,0.805282774523917,-0.667600711484946));
#9948=CARTESIAN_POINT('Ctrl Pts',(0.544416813021393,0.803352493165594,-0.664841874904024));
#9949=CARTESIAN_POINT('Ctrl Pts',(0.778500733721097,0.804617356522799,-0.666707630946455));
#9950=CARTESIAN_POINT('Ctrl Pts',(1.10459149410625,0.804732922624886,-0.666877921514692));
#9951=CARTESIAN_POINT('Ctrl Pts',(1.51421516428224,0.804089532801427,-0.665931138084407));
#9952=CARTESIAN_POINT('Ctrl Pts',(1.83620821687538,0.804649660698633,-0.66675251787415));
#9953=CARTESIAN_POINT('Ctrl Pts',(2.00015071794412,0.804475523135573,-0.666497406911305));
#9954=CARTESIAN_POINT('',(2.00009323767342,0.735984691360175,-0.676310263121555));
#9955=CARTESIAN_POINT('Origin',(1.99999999999998,0.759999999999999,-0.60000000000007));
#9956=CARTESIAN_POINT('',(0.600124355483127,-0.0799998580128369,-2.00008516830249));
#9957=CARTESIAN_POINT('Ctrl Pts',(0.600124355483126,-0.0799998580128369,
-2.00008516830249));
#9958=CARTESIAN_POINT('Ctrl Pts',(0.600379376695518,-0.0801739343158842,
-1.83620033785433));
#9959=CARTESIAN_POINT('Ctrl Pts',(0.599562611053881,-0.0796184124528264,
-1.5144754520526));
#9960=CARTESIAN_POINT('Ctrl Pts',(0.600502518404447,-0.0802525034314073,
-1.10424411057565));
#9961=CARTESIAN_POINT('Ctrl Pts',(0.600344602427935,-0.0801506833161176,
-0.778901942331774));
#9962=CARTESIAN_POINT('Ctrl Pts',(0.598456953704134,-0.0788587712934794,
-0.544242160533997));
#9963=CARTESIAN_POINT('Ctrl Pts',(0.601272474507003,-0.0808543685860998,
-0.287680267082095));
#9964=CARTESIAN_POINT('Ctrl Pts',(0.605184477979747,-0.0824681761820383,
-0.0307556431383126));
#9965=CARTESIAN_POINT('Ctrl Pts',(0.588609512632607,-0.0742202560328195,
0.161001223625551));
#9966=CARTESIAN_POINT('Ctrl Pts',(0.518063450209372,-0.0648906358873938,
0.323627369018429));
#9967=CARTESIAN_POINT('Ctrl Pts',(0.389740128736442,-0.0579722786893707,
0.474748184678881));
#9968=CARTESIAN_POINT('Ctrl Pts',(0.173020606908044,-0.0467144436845919,
0.602178110487582));
#9969=CARTESIAN_POINT('Ctrl Pts',(-0.156647509262585,-0.0336993466160229,
0.628366170043479));
#9970=CARTESIAN_POINT('Ctrl Pts',(-0.534302969503257,-0.01563383198389,
0.396152535345114));
#9971=CARTESIAN_POINT('Ctrl Pts',(-0.680181221263981,0.00400588873282267,
-0.0887030397692518));
#9972=CARTESIAN_POINT('Ctrl Pts',(-0.465603142330848,0.0202821362637637,
-0.446134214125788));
#9973=CARTESIAN_POINT('Ctrl Pts',(-0.165486932860075,0.03474270768116,-0.612245575240685));
#9974=CARTESIAN_POINT('Ctrl Pts',(0.146295095787791,0.0474352484480225,
-0.642641412885972));
#9975=CARTESIAN_POINT('Ctrl Pts',(0.495949774692522,0.0637997238881112,
-0.436123139243827));
#9976=CARTESIAN_POINT('Ctrl Pts',(0.659385538859151,0.0802233041204479,
-0.0644782106763051));
#9977=CARTESIAN_POINT('Ctrl Pts',(0.574545201045043,0.0966991572901908,
0.334449484668907));
#9978=CARTESIAN_POINT('Ctrl Pts',(0.271532605139402,0.113229721085999,0.609171048717871));
#9979=CARTESIAN_POINT('Ctrl Pts',(-0.136251969463658,0.129813195665052,
0.654997123118035));
#9980=CARTESIAN_POINT('Ctrl Pts',(-0.494901592911036,0.146449576154649,
0.453502429895765));
#9981=CARTESIAN_POINT('Ctrl Pts',(-0.668917284177339,0.163138203343486,
0.0782620703516101));
#9982=CARTESIAN_POINT('Ctrl Pts',(-0.598644996586867,0.178018517289954,
-0.282046799603755));
#9983=CARTESIAN_POINT('Ctrl Pts',(-0.335262243900907,0.194801447000121,
-0.590258574308657));
#9984=CARTESIAN_POINT('Ctrl Pts',(0.0833281156314849,0.211635077569448,
-0.691395156339746));
#9985=CARTESIAN_POINT('Ctrl Pts',(0.4320119853653,0.227588446215705,-0.502587368796631));
#9986=CARTESIAN_POINT('Ctrl Pts',(0.58527223262087,0.238874211068699,-0.281979562605746));
#9987=CARTESIAN_POINT('Ctrl Pts',(0.678917739338141,0.252059849462334,0.0184388692246381));
#9988=CARTESIAN_POINT('Ctrl Pts',(0.554821413577227,0.270001502682695,0.463024783480917));
#9989=CARTESIAN_POINT('Ctrl Pts',(0.089888824047859,0.290221470828933,0.693551038003489));
#9990=CARTESIAN_POINT('Ctrl Pts',(-0.272915151999609,0.305432097922516,
0.607393400489082));
#9991=CARTESIAN_POINT('Ctrl Pts',(-0.465626168527264,0.315590515005467,
0.46173311346713));
#9992=CARTESIAN_POINT('Ctrl Pts',(-0.611423927492396,0.325760833794014,
0.268821318511434));
#9993=CARTESIAN_POINT('Ctrl Pts',(-0.698650473779508,0.341042831595186,
-0.0956472554953462));
#9994=CARTESIAN_POINT('Ctrl Pts',(-0.465321982498693,0.361476665326508,
-0.565350807747607));
#9995=CARTESIAN_POINT('Ctrl Pts',(0.10575120321005,0.38454069790763,-0.726974188805798));
#9996=CARTESIAN_POINT('Ctrl Pts',(0.610387251745808,0.407678360873112,-0.412408779209339));
#9997=CARTESIAN_POINT('Ctrl Pts',(0.718323895495084,0.430887045922702,0.17413060542287));
#9998=CARTESIAN_POINT('Ctrl Pts',(0.355237119019683,0.454164351458316,0.650683811024646));
#9999=CARTESIAN_POINT('Ctrl Pts',(-0.175382406590221,0.4749142230429,0.695878649309196));
#10000=CARTESIAN_POINT('Ctrl Pts',(-0.54101475967607,0.49311138275633,0.440269492223299));
#10001=CARTESIAN_POINT('Ctrl Pts',(-0.693527526572458,0.50873629806685,
0.0898379898580044));
#10002=CARTESIAN_POINT('Ctrl Pts',(-0.646735970560938,0.521779183073869,
-0.226461651899009));
#10003=CARTESIAN_POINT('Ctrl Pts',(-0.513906112786406,0.532226370805735,
-0.436433419735239));
#10004=CARTESIAN_POINT('Ctrl Pts',(-0.328920782360512,0.542681936352062,
-0.602852159734885));
#10005=CARTESIAN_POINT('Ctrl Pts',(-0.0243494995865983,0.55576702001899,
-0.701905622444322));
#10006=CARTESIAN_POINT('Ctrl Pts',(0.318684360355662,0.570182439320145,
-0.618057422392217));
#10007=CARTESIAN_POINT('Ctrl Pts',(0.554275268889935,0.583304705413154,
-0.407908493988256));
#10008=CARTESIAN_POINT('Ctrl Pts',(0.713586310862138,0.599067032359038,
-0.0629718800249659));
#10009=CARTESIAN_POINT('Ctrl Pts',(0.617323759198901,0.61880473745743,0.433855029903579));
#10010=CARTESIAN_POINT('Ctrl Pts',(0.0931818027763926,0.642526983889894,
0.749181117386836));
#10011=CARTESIAN_POINT('Ctrl Pts',(-0.314313763037281,0.659133011706964,
0.627311226200405));
#10012=CARTESIAN_POINT('Ctrl Pts',(-0.477269723836412,0.668539639010893,
0.476341934975343));
#10013=CARTESIAN_POINT('Ctrl Pts',(-0.524957853949116,0.671513213020625,
0.424882768662061));
#10014=CARTESIAN_POINT('Ctrl Pts',(-0.597179322807005,0.676677358782867,
0.325569816011966));
#10015=CARTESIAN_POINT('Ctrl Pts',(-0.69448376569806,0.6873032670482,0.0964041117283874));
#10016=CARTESIAN_POINT('Ctrl Pts',(-0.671478747098358,0.69869719950028,
-0.197322255866813));
#10017=CARTESIAN_POINT('Ctrl Pts',(-0.527686488423399,0.711441182605667,
-0.440569074748579));
#10018=CARTESIAN_POINT('Ctrl Pts',(-0.36114955668007,0.719020822056164,
-0.583433135906584));
#10019=CARTESIAN_POINT('Ctrl Pts',(-0.171544666302877,0.729888896055897,
-0.664752607658936));
#10020=CARTESIAN_POINT('Ctrl Pts',(0.0327819626725445,0.738541246775484,
-0.681326463162123));
#10021=CARTESIAN_POINT('Ctrl Pts',(0.287281763425397,0.736796378226309,
-0.677467579294977));
#10022=CARTESIAN_POINT('Ctrl Pts',(0.544477498698488,0.734860197456536,
-0.674632411152923));
#10023=CARTESIAN_POINT('Ctrl Pts',(0.778765801010588,0.736127346477361,
-0.676530344298986));
#10024=CARTESIAN_POINT('Ctrl Pts',(1.10435275137728,0.736241519844584,-0.676684603908725));
#10025=CARTESIAN_POINT('Ctrl Pts',(1.51439530422594,0.735599108498541,-0.675749139626198));
#10026=CARTESIAN_POINT('Ctrl Pts',(1.83620130898864,0.736158775205915,-0.676565295388702));
#10027=CARTESIAN_POINT('Ctrl Pts',(2.00009323767342,0.735984691360175,-0.676310263121555));
#10028=CARTESIAN_POINT('Origin',(0.6,0.,-2.));
#10029=CARTESIAN_POINT('Ctrl Pts',(0.528325516000818,0.0355351383793534,
-1.99985072236852));
#10030=CARTESIAN_POINT('Ctrl Pts',(0.528580216238454,0.0353612811721935,
-1.83617216061816));
#10031=CARTESIAN_POINT('Ctrl Pts',(0.527763128960968,0.0359074110765236,
-1.51524836790432));
#10032=CARTESIAN_POINT('Ctrl Pts',(0.52869398879819,0.0352930571869228,
-1.10323975855771));
#10033=CARTESIAN_POINT('Ctrl Pts',(0.528539994622404,0.0353667487690795,
-0.780063536259368));
#10034=CARTESIAN_POINT('Ctrl Pts',(0.52663921660727,0.0367139095688948,
-0.544390644686365));
#10035=CARTESIAN_POINT('Ctrl Pts',(0.529476659613029,0.034585865490992,
-0.284703947187213));
#10036=CARTESIAN_POINT('Ctrl Pts',(0.533317427829506,0.0332656496173089,
-0.0318821597569514));
#10037=CARTESIAN_POINT('Ctrl Pts',(0.520047835906791,0.03934019911185,0.11127177591819));
#10038=CARTESIAN_POINT('Ctrl Pts',(0.487979861380134,0.0447394305988247,
0.206368682333952));
#10039=CARTESIAN_POINT('Ctrl Pts',(0.43700205055529,0.0496761629927893,
0.303336604975879));
#10040=CARTESIAN_POINT('Ctrl Pts',(0.343595116172016,0.0549025285724336,
0.412156142305733));
#10041=CARTESIAN_POINT('Ctrl Pts',(0.155413324632073,0.0645663572156617,
0.523171635285862));
#10042=CARTESIAN_POINT('Ctrl Pts',(-0.13238197811405,0.0760053922841299,
0.546096961811003));
#10043=CARTESIAN_POINT('Ctrl Pts',(-0.458547546709041,0.0915759716479705,
0.344626269173423));
#10044=CARTESIAN_POINT('Ctrl Pts',(-0.583900979357653,0.108513502601817,
-0.0726418166757439));
#10045=CARTESIAN_POINT('Ctrl Pts',(-0.399874479395914,0.122418645633365,
-0.378151431589044));
#10046=CARTESIAN_POINT('Ctrl Pts',(-0.144208713332262,0.134741070398731,
-0.519625470017589));
#10047=CARTESIAN_POINT('Ctrl Pts',(0.120678163831248,0.145520914168386,
-0.545280477556419));
#10048=CARTESIAN_POINT('Ctrl Pts',(0.416245026241475,0.159362036169617,
-0.370399044184566));
#10049=CARTESIAN_POINT('Ctrl Pts',(0.553682940345137,0.173192726374506,
-0.0573370873951302));
#10050=CARTESIAN_POINT('Ctrl Pts',(0.482308934415198,0.187011877340453,
0.277215748417183));
#10051=CARTESIAN_POINT('Ctrl Pts',(0.229028777221665,0.200821622625116,
0.506563345532159));
#10052=CARTESIAN_POINT('Ctrl Pts',(-0.110367911292249,0.214623077889557,
0.54450512639393));
#10053=CARTESIAN_POINT('Ctrl Pts',(-0.407671943899019,0.228418134002614,
0.377255910602494));
#10054=CARTESIAN_POINT('Ctrl Pts',(-0.551281224571261,0.242207799546803,
0.0671237295171103));
#10055=CARTESIAN_POINT('Ctrl Pts',(-0.493275743670343,0.254462041472817,
-0.229567370520871));
#10056=CARTESIAN_POINT('Ctrl Pts',(-0.276873119070605,0.268246207770326,
-0.482655650599567));
#10057=CARTESIAN_POINT('Ctrl Pts',(0.0659203358970661,0.282029146223394,
-0.565205026128377));
#10058=CARTESIAN_POINT('Ctrl Pts',(0.350357710654226,0.295047091504507,
-0.410999506466758));
#10059=CARTESIAN_POINT('Ctrl Pts',(0.475135516148999,0.304237345274322,
-0.231346154144024));
#10060=CARTESIAN_POINT('Ctrl Pts',(0.551288205940918,0.314960561464671,
0.0129747269886634));
#10061=CARTESIAN_POINT('Ctrl Pts',(0.45022254899038,0.329517029083473,0.37370896603078));
#10062=CARTESIAN_POINT('Ctrl Pts',(0.0742959024516958,0.345869925490746,
0.559751696715401));
#10063=CARTESIAN_POINT('Ctrl Pts',(-0.267515912073187,0.360187665470484,
0.478838803845945));
#10064=CARTESIAN_POINT('Ctrl Pts',(-0.479551721793889,0.372466952348416,
0.266530966916759));
#10065=CARTESIAN_POINT('Ctrl Pts',(-0.561020874450445,0.386802304141767,
-0.0756540266283994));
#10066=CARTESIAN_POINT('Ctrl Pts',(-0.373798964410677,0.40320076690853,
-0.452338944214845));
#10067=CARTESIAN_POINT('Ctrl Pts',(0.0837095501434262,0.421672873429502,
-0.581681018186793));
#10068=CARTESIAN_POINT('Ctrl Pts',(0.487056597627596,0.440172228021392,
-0.33000386321063));
#10069=CARTESIAN_POINT('Ctrl Pts',(0.573129832954481,0.458702467353384,
0.138301209287518));
#10070=CARTESIAN_POINT('Ctrl Pts',(0.283467753989205,0.477266746895905,
0.518306234712299));
#10071=CARTESIAN_POINT('Ctrl Pts',(-0.139343171325179,0.49380124199818,
0.554254940466149));
#10072=CARTESIAN_POINT('Ctrl Pts',(-0.430585233273848,0.508295268221301,
0.350657311113887));
#10073=CARTESIAN_POINT('Ctrl Pts',(-0.551985372269875,0.520737714298862,
0.0715900336355947));
#10074=CARTESIAN_POINT('Ctrl Pts',(-0.507419925273811,0.533200036247129,
-0.230607774684784));
#10075=CARTESIAN_POINT('Ctrl Pts',(-0.31033354343041,0.545683195018118,
-0.464206836172492));
#10076=CARTESIAN_POINT('Ctrl Pts',(-0.0190318124706425,0.55818804173365,
-0.558876538153605));
#10077=CARTESIAN_POINT('Ctrl Pts',(0.253983768099081,0.569671725898546,
-0.492060874631647));
#10078=CARTESIAN_POINT('Ctrl Pts',(0.442244523118364,0.580128296331906,
-0.324658610947337));
#10079=CARTESIAN_POINT('Ctrl Pts',(0.520722105088888,0.587982684618036,
-0.152670499369794));
#10080=CARTESIAN_POINT('Ctrl Pts',(0.546710027901627,0.597417021784907,
0.0692065446470551));
#10081=CARTESIAN_POINT('Ctrl Pts',(0.456423583474616,0.610019390825592,
0.367751194847143));
#10082=CARTESIAN_POINT('Ctrl Pts',(0.0741878943616268,0.627382577648326,
0.598649005107442));
#10083=CARTESIAN_POINT('Ctrl Pts',(-0.252446137124855,0.640668092490499,
0.501260226779611));
#10084=CARTESIAN_POINT('Ctrl Pts',(-0.382734909615739,0.648193686386572,
0.380473706897257));
#10085=CARTESIAN_POINT('Ctrl Pts',(-0.42091088190008,0.650570748345437,
0.339327536657439));
#10086=CARTESIAN_POINT('Ctrl Pts',(-0.478799050747207,0.654727247608708,
0.259486984260798));
#10087=CARTESIAN_POINT('Ctrl Pts',(-0.557131063499655,0.663174776823465,
0.0765261952556552));
#10088=CARTESIAN_POINT('Ctrl Pts',(-0.537566049825482,0.672499456879064,
-0.160776378174217));
#10089=CARTESIAN_POINT('Ctrl Pts',(-0.423528711452778,0.682478562361745,
-0.354330430488681));
#10090=CARTESIAN_POINT('Ctrl Pts',(-0.311592387005274,0.687842301956471,
-0.450400927405352));
#10091=CARTESIAN_POINT('Ctrl Pts',(-0.211665405946688,0.692933513783124,
-0.502993006931043));
#10092=CARTESIAN_POINT('Ctrl Pts',(-0.112852189303309,0.69854100703458,
-0.536239978733061));
#10093=CARTESIAN_POINT('Ctrl Pts',(0.0321928148234355,0.704663557813275,
-0.549477537118094));
#10094=CARTESIAN_POINT('Ctrl Pts',(0.28467574209202,0.703327852119614,-0.545661762520716));
#10095=CARTESIAN_POINT('Ctrl Pts',(0.544418006349421,0.701207276752475,
-0.542811541675268));
#10096=CARTESIAN_POINT('Ctrl Pts',(0.780045344880861,0.702551643433085,
-0.544716466237711));
#10097=CARTESIAN_POINT('Ctrl Pts',(1.10325708111259,0.702626966137619,-0.544867419416464));
#10098=CARTESIAN_POINT('Ctrl Pts',(1.5152368295222,0.70201184590394,-0.543937156859423));
#10099=CARTESIAN_POINT('Ctrl Pts',(1.83617236681158,0.702558621549799,-0.544752786768393));
#10100=CARTESIAN_POINT('Ctrl Pts',(1.9998524353109,0.702384762739154,-0.544498084176928));
#10101=CARTESIAN_POINT('Ctrl Pts',(0.518006988619909,0.0147226621587207,
-1.99985677244376));
#10102=CARTESIAN_POINT('Ctrl Pts',(0.51826169653407,0.0145487997116001,
-1.83617327751152));
#10103=CARTESIAN_POINT('Ctrl Pts',(0.517439258498296,0.0150951255434231,
-1.51522865062124));
#10104=CARTESIAN_POINT('Ctrl Pts',(0.518364404194574,0.0144817764415016,
-1.10324322288189));
#10105=CARTESIAN_POINT('Ctrl Pts',(0.518203712856234,0.0145552635795002,
-0.780023366489656));
#10106=CARTESIAN_POINT('Ctrl Pts',(0.516302146489189,0.0159040910419349,
-0.544343077372114));
#10107=CARTESIAN_POINT('Ctrl Pts',(0.519119939486031,0.0137739026997169,
-0.284772538321969));
#10108=CARTESIAN_POINT('Ctrl Pts',(0.522975085576804,0.0124609380717381,
-0.0315732326310645));
#10109=CARTESIAN_POINT('Ctrl Pts',(0.509643674692382,0.018517597343244,
0.110651199452232));
#10110=CARTESIAN_POINT('Ctrl Pts',(0.47832511502757,0.0237806788581772,
0.203319306803046));
#10111=CARTESIAN_POINT('Ctrl Pts',(0.428443867571616,0.028616054359568,
0.29829212926619));
#10112=CARTESIAN_POINT('Ctrl Pts',(0.336639314786772,0.033752976935528,
0.405215900979145));
#10113=CARTESIAN_POINT('Ctrl Pts',(0.151994665964955,0.0432358978067775,
0.514121724925737));
#10114=CARTESIAN_POINT('Ctrl Pts',(-0.130966602912282,0.0544866325216903,
0.536764222009815));
#10115=CARTESIAN_POINT('Ctrl Pts',(-0.451809607501558,0.0698051303173712,
0.338584434964127));
#10116=CARTESIAN_POINT('Ctrl Pts',(-0.575501058572054,0.0864976418736099,
-0.072428206504078));
#10117=CARTESIAN_POINT('Ctrl Pts',(-0.394000818625767,0.100217666459796,
-0.373861821833153));
#10118=CARTESIAN_POINT('Ctrl Pts',(-0.141611300945278,0.112384059902738,
-0.513558715621065));
#10119=CARTESIAN_POINT('Ctrl Pts',(0.120151382692751,0.123039230651802,
-0.538926981640901));
#10120=CARTESIAN_POINT('Ctrl Pts',(0.412599084171835,0.136736320530498,
-0.365982567622163));
#10121=CARTESIAN_POINT('Ctrl Pts',(0.548778764164466,0.150437544146518,
-0.0559340071012521));
#10122=CARTESIAN_POINT('Ctrl Pts',(0.478069875663281,0.164143621167663,
0.275811473392926));
#10123=CARTESIAN_POINT('Ctrl Pts',(0.226673355209394,0.177856074698083,
0.503539697370229));
#10124=CARTESIAN_POINT('Ctrl Pts',(-0.110644606215152,0.191576390642706,
0.541311737028743));
#10125=CARTESIAN_POINT('Ctrl Pts',(-0.406509930397425,0.20530665826345,
0.374938573118697));
#10126=CARTESIAN_POINT('Ctrl Pts',(-0.549639073980249,0.219047557375228,
0.0659995113422246));
#10127=CARTESIAN_POINT('Ctrl Pts',(-0.491828299868531,0.231273972126515,
-0.229959181959865));
#10128=CARTESIAN_POINT('Ctrl Pts',(-0.27580622579465,0.245037965029692,
-0.482642962691277));
#10129=CARTESIAN_POINT('Ctrl Pts',(0.0667891693692878,0.258815642204134,
-0.56526745809795));
#10130=CARTESIAN_POINT('Ctrl Pts',(0.351583495751141,0.271851711458274,
-0.41095497024062));
#10131=CARTESIAN_POINT('Ctrl Pts',(0.476585714824317,0.281058974417471,
-0.230992328401952));
#10132=CARTESIAN_POINT('Ctrl Pts',(0.552929626102851,0.291807850647884,
0.0138816394099051));
#10133=CARTESIAN_POINT('Ctrl Pts',(0.451593915839779,0.306425020358756,
0.375986515342406));
#10134=CARTESIAN_POINT('Ctrl Pts',(0.0738204095193084,0.322862572045568,
0.563103116958926));
#10135=CARTESIAN_POINT('Ctrl Pts',(-0.270167738435555,0.337272921272754,
0.481717326921321));
#10136=CARTESIAN_POINT('Ctrl Pts',(-0.483806774332006,0.349644528947839,
0.267882725040153));
#10137=CARTESIAN_POINT('Ctrl Pts',(-0.56600730933755,0.364102175236501,
-0.0771625257846216));
#10138=CARTESIAN_POINT('Ctrl Pts',(-0.377092271910289,0.380665601055743,
-0.457594185300374));
#10139=CARTESIAN_POINT('Ctrl Pts',(0.0855089279844419,0.399348369251059,
-0.588538803959294));
#10140=CARTESIAN_POINT('Ctrl Pts',(0.494066616980439,0.418086689130485,
-0.333792905023513));
#10141=CARTESIAN_POINT('Ctrl Pts',(0.581499054249072,0.436883611950722,
0.1411231143738));
#10142=CARTESIAN_POINT('Ctrl Pts',(0.287433008810201,0.455740676787563,
0.527163124276987));
#10143=CARTESIAN_POINT('Ctrl Pts',(-0.142615978537236,0.47256294829645,
0.563831621580814));
#10144=CARTESIAN_POINT('Ctrl Pts',(-0.439170122070614,0.487320513166624,
0.356588512723425));
#10145=CARTESIAN_POINT('Ctrl Pts',(-0.562904282860289,0.500001367061856,
0.0722157106208628));
#10146=CARTESIAN_POINT('Ctrl Pts',(-0.517490882361781,0.512715724688964,
-0.236051271509166));
#10147=CARTESIAN_POINT('Ctrl Pts',(-0.316295712666788,0.5254626426108,-0.474559379294206));
#10148=CARTESIAN_POINT('Ctrl Pts',(-0.0186872380461836,0.538239998427524,
-0.571332456617058));
#10149=CARTESIAN_POINT('Ctrl Pts',(0.260497964274366,0.549984096113616,
-0.503029943852036));
#10150=CARTESIAN_POINT('Ctrl Pts',(0.453172437169254,0.560685984855627,
-0.331743989022342));
#10151=CARTESIAN_POINT('Ctrl Pts',(0.533542764846318,0.568729832734574,
-0.155636638327312));
#10152=CARTESIAN_POINT('Ctrl Pts',(0.56017130075111,0.578393043619417,0.0716182619860427));
#10153=CARTESIAN_POINT('Ctrl Pts',(0.467665246161068,0.591312818479437,
0.377633597364541));
#10154=CARTESIAN_POINT('Ctrl Pts',(0.0755416097489565,0.609130487126725,
0.614648364140295));
#10155=CARTESIAN_POINT('Ctrl Pts',(-0.25999452114002,0.622779933154743,
0.514691601607703));
#10156=CARTESIAN_POINT('Ctrl Pts',(-0.393897285477323,0.630514235023044,
0.390563383963501));
#10157=CARTESIAN_POINT('Ctrl Pts',(-0.433131000099862,0.632957419536418,
0.34827185345534));
#10158=CARTESIAN_POINT('Ctrl Pts',(-0.492626078021695,0.637228232855216,
0.266240605920182));
#10159=CARTESIAN_POINT('Ctrl Pts',(-0.573128984843918,0.64591806968787,
0.0780451747198588));
#10160=CARTESIAN_POINT('Ctrl Pts',(-0.553160666421587,0.655505290269903,
-0.165943772968861));
#10161=CARTESIAN_POINT('Ctrl Pts',(-0.43559455019087,0.665789433238246,
-0.365425437099108));
#10162=CARTESIAN_POINT('Ctrl Pts',(-0.320468157151283,0.671307222232064,
-0.464218402012083));
#10163=CARTESIAN_POINT('Ctrl Pts',(-0.217516188562935,0.676551531702204,
-0.518462754427448));
#10164=CARTESIAN_POINT('Ctrl Pts',(-0.114896708172773,0.682375360770741,
-0.552926885225282));
#10165=CARTESIAN_POINT('Ctrl Pts',(0.0324089213706158,0.68855646510286,
-0.566177806035642));
#10166=CARTESIAN_POINT('Ctrl Pts',(0.284694547996705,0.68720379020063,-0.562380851818847));
#10167=CARTESIAN_POINT('Ctrl Pts',(0.544416635062839,0.685091793638103,
-0.559529116763886));
#10168=CARTESIAN_POINT('Ctrl Pts',(0.779973909884199,0.686433174919341,
-0.561439259023152));
#10169=CARTESIAN_POINT('Ctrl Pts',(1.10328957662273,0.686510451152178,-0.561591177867606));
#10170=CARTESIAN_POINT('Ctrl Pts',(1.51519744302046,0.685894630299126,-0.560665320718706));
#10171=CARTESIAN_POINT('Ctrl Pts',(1.83617381496558,0.686442247831574,-0.561482812535836));
#10172=CARTESIAN_POINT('Ctrl Pts',(1.99986135028159,0.686268381089775,-0.561228098325256));
#10173=CARTESIAN_POINT('Ctrl Pts',(0.517064965384546,-0.0276174348744286,
-1.99990027965328));
#10174=CARTESIAN_POINT('Ctrl Pts',(0.517319733648456,-0.0277913385160093,
-1.83617800203207));
#10175=CARTESIAN_POINT('Ctrl Pts',(0.516501154978697,-0.0272448942899652,
-1.51509441856937));
#10176=CARTESIAN_POINT('Ctrl Pts',(0.517439825994783,-0.0278604744543955,
-1.10345697185989));
#10177=CARTESIAN_POINT('Ctrl Pts',(0.51727868303505,-0.0277855206568046,
-0.779843367061392));
#10178=CARTESIAN_POINT('Ctrl Pts',(0.515395748265278,-0.0264409292158762,
-0.544362732023317));
#10179=CARTESIAN_POINT('Ctrl Pts',(0.518196318364542,-0.0285631971806174,
-0.285399374400077));
#10180=CARTESIAN_POINT('Ctrl Pts',(0.522130009157292,-0.0298969535989713,
-0.0312837912576946));
#10181=CARTESIAN_POINT('Ctrl Pts',(0.508630669142978,-0.0237744096040658,
0.11273833187974));
#10182=CARTESIAN_POINT('Ctrl Pts',(0.477303002332513,-0.0185175895096401,
0.205186241209719));
#10183=CARTESIAN_POINT('Ctrl Pts',(0.42771780622717,-0.0137076224884299,
0.299712541386803));
#10184=CARTESIAN_POINT('Ctrl Pts',(0.335710255161657,-0.00855651946997313,
0.406906376567326));
#10185=CARTESIAN_POINT('Ctrl Pts',(0.150598154466753,0.000948902484060557,
0.516127151823611));
#10186=CARTESIAN_POINT('Ctrl Pts',(-0.133196632035283,0.0122299278698042,
0.538860692452965));
#10187=CARTESIAN_POINT('Ctrl Pts',(-0.456043768540289,0.0276354505277528,
0.339704505103172));
#10188=CARTESIAN_POINT('Ctrl Pts',(-0.580879226861971,0.0444564053811016,
-0.0746224708782053));
#10189=CARTESIAN_POINT('Ctrl Pts',(-0.397598943967096,0.0583258466825628,
-0.379524117797193));
#10190=CARTESIAN_POINT('Ctrl Pts',(-0.141860962022226,0.0706512785723848,
-0.52105662949048));
#10191=CARTESIAN_POINT('Ctrl Pts',(0.123618324751229,0.0814558379837331,
-0.546900551930632));
#10192=CARTESIAN_POINT('Ctrl Pts',(0.420944460563251,0.0953736393877776,
-0.371199562504824));
#10193=CARTESIAN_POINT('Ctrl Pts',(0.55975828999923,0.10932616565685,-0.0554275481068647));
#10194=CARTESIAN_POINT('Ctrl Pts',(0.487690702846842,0.123311797342578,
0.283210359890105));
#10195=CARTESIAN_POINT('Ctrl Pts',(0.230638240284097,0.137332741277447,
0.516210623580482));
#10196=CARTESIAN_POINT('Ctrl Pts',(-0.115050726500188,0.151389888098985,
0.555028062340877));
#10197=CARTESIAN_POINT('Ctrl Pts',(-0.418919310186353,0.165484870541764,
0.384283721259028));
#10198=CARTESIAN_POINT('Ctrl Pts',(-0.566287603572425,0.179618646099089,
0.0664636290862337));
#10199=CARTESIAN_POINT('Ctrl Pts',(-0.506778045012059,0.192217438048822,
-0.238621244470182));
#10200=CARTESIAN_POINT('Ctrl Pts',(-0.283781109838095,0.206426241219143,
-0.49957208381572));
#10201=CARTESIAN_POINT('Ctrl Pts',(0.0706066034421951,0.220677604075878,
-0.585193411698452));
#10202=CARTESIAN_POINT('Ctrl Pts',(0.365832693978764,0.234183813926373,
-0.42534652150558));
#10203=CARTESIAN_POINT('Ctrl Pts',(0.495619738153408,0.243741154450391,
-0.238511686590906));
#10204=CARTESIAN_POINT('Ctrl Pts',(0.57495990921569,0.254909247382493,0.0159208359312727));
#10205=CARTESIAN_POINT('Ctrl Pts',(0.469740551468291,0.270107361335315,
0.392695173251977));
#10206=CARTESIAN_POINT('Ctrl Pts',(0.0757962012645511,0.287249204171579,
0.588020269692376));
#10207=CARTESIAN_POINT('Ctrl Pts',(-0.283683402920196,0.302304485175122,
0.503073075011702));
#10208=CARTESIAN_POINT('Ctrl Pts',(-0.507263064087155,0.315247977872081,
0.279334514400664));
#10209=CARTESIAN_POINT('Ctrl Pts',(-0.593480268797605,0.330395219740859,
-0.0821951824371391));
#10210=CARTESIAN_POINT('Ctrl Pts',(-0.395345834233177,0.34777246937306,
-0.481527416128932));
#10211=CARTESIAN_POINT('Ctrl Pts',(0.091088459307557,0.367415692906852,
-0.619429636770056));
#10212=CARTESIAN_POINT('Ctrl Pts',(0.521654838632725,0.387153663215753,
-0.351178853221841));
#10213=CARTESIAN_POINT('Ctrl Pts',(0.614127000564708,0.406988410964741,
0.150060798600657));
#10214=CARTESIAN_POINT('Ctrl Pts',(0.303351339173566,0.426921933914876,
0.558318532423771));
#10215=CARTESIAN_POINT('Ctrl Pts',(-0.15200412641022,0.444728306814291,
0.597312366353538));
#10216=CARTESIAN_POINT('Ctrl Pts',(-0.46651007651178,0.460376324275656,
0.377578786974955));
#10217=CARTESIAN_POINT('Ctrl Pts',(-0.597896215312271,0.473834148081358,
0.0757644518309022));
#10218=CARTESIAN_POINT('Ctrl Pts',(-0.549688991211359,0.487337171079593,
-0.251696035827126));
#10219=CARTESIAN_POINT('Ctrl Pts',(-0.33582481262013,0.500886334893807,
-0.505310469715122));
#10220=CARTESIAN_POINT('Ctrl Pts',(-0.0191083072298206,0.51448271913657,
-0.608315954390084));
#10221=CARTESIAN_POINT('Ctrl Pts',(0.278244251614214,0.526989032687595,
-0.535616391608276));
#10222=CARTESIAN_POINT('Ctrl Pts',(0.483576818183559,0.538392269039443,
-0.353074191952224));
#10223=CARTESIAN_POINT('Ctrl Pts',(0.569283164476684,0.546967375765335,
-0.1653038864453));
#10224=CARTESIAN_POINT('Ctrl Pts',(0.597681099378553,0.557277057685444,
0.0771548913991258));
#10225=CARTESIAN_POINT('Ctrl Pts',(0.499022954209422,0.571061850450283,
0.403754875104057));
#10226=CARTESIAN_POINT('Ctrl Pts',(0.0801878602785286,0.59009117728441,
0.656954926766208));
#10227=CARTESIAN_POINT('Ctrl Pts',(-0.278435050767254,0.604675594610773,
0.550184775122633));
#10228=CARTESIAN_POINT('Ctrl Pts',(-0.421702877060122,0.612949989901589,
0.417381582961095));
#10229=CARTESIAN_POINT('Ctrl Pts',(-0.463678194708879,0.615564544680876,
0.372121041656761));
#10230=CARTESIAN_POINT('Ctrl Pts',(-0.527311587821278,0.62012833630386,
0.284465723612475));
#10231=CARTESIAN_POINT('Ctrl Pts',(-0.613338062910082,0.62943639172353,
0.0828777024836109));
#10232=CARTESIAN_POINT('Ctrl Pts',(-0.592374455216482,0.639666807274975,
-0.177632373915939));
#10233=CARTESIAN_POINT('Ctrl Pts',(-0.465998063899403,0.650709650428148,
-0.391877889696578));
#10234=CARTESIAN_POINT('Ctrl Pts',(-0.342932122259441,0.656609679460992,
-0.497401597437851));
#10235=CARTESIAN_POINT('Ctrl Pts',(-0.232874147112921,0.662211754394164,
-0.555492407774234));
#10236=CARTESIAN_POINT('Ctrl Pts',(-0.121097630640796,0.668559783851406,
-0.592927928496883));
#10237=CARTESIAN_POINT('Ctrl Pts',(0.0328311030844529,0.674923577641489,
-0.606297423549468));
#10238=CARTESIAN_POINT('Ctrl Pts',(0.285189029776664,0.673515276722222,
-0.602484355047046));
#10239=CARTESIAN_POINT('Ctrl Pts',(0.544464931121522,0.671428302466708,
-0.599629698570021));
#10240=CARTESIAN_POINT('Ctrl Pts',(0.779716204754393,0.672759167364569,
-0.601534551529286));
#10241=CARTESIAN_POINT('Ctrl Pts',(1.10352456500245,0.672841678894774,-0.60168402557845));
#10242=CARTESIAN_POINT('Ctrl Pts',(1.51502500132075,0.67222198428823,-0.600751926240327));
#10243=CARTESIAN_POINT('Ctrl Pts',(1.83617907898506,0.672771254551909,-0.601566211172317));
#10244=CARTESIAN_POINT('Ctrl Pts',(1.99990920276725,0.672597342573202,-0.601311430689815));
#10245=CARTESIAN_POINT('Ctrl Pts',(0.553753009580757,-0.0708264141617583,
-2.00000326593235));
#10246=CARTESIAN_POINT('Ctrl Pts',(0.554007918554055,-0.0710004138509187,
-1.83619056393385));
#10247=CARTESIAN_POINT('Ctrl Pts',(0.553185359331648,-0.0704511009669655,
-1.51473935544524));
#10248=CARTESIAN_POINT('Ctrl Pts',(0.554128520828115,-0.0710714148493772,
-1.10390624361236));
#10249=CARTESIAN_POINT('Ctrl Pts',(0.55395750433957,-0.0709884976154986,
-0.779299644098123));
#10250=CARTESIAN_POINT('Ctrl Pts',(0.552089915743917,-0.0696580104253656,
-0.544343141096708));
#10251=CARTESIAN_POINT('Ctrl Pts',(0.554847476208613,-0.0717441098715436,
-0.286553871632578));
#10252=CARTESIAN_POINT('Ctrl Pts',(0.558871807050512,-0.0731549107076979,
-0.0311242532742824));
#10253=CARTESIAN_POINT('Ctrl Pts',(0.544996993740645,-0.06677124873102,
0.121479781678294));
#10254=CARTESIAN_POINT('Ctrl Pts',(0.510876588740922,-0.0610344785127724,
0.222168271083783));
#10255=CARTESIAN_POINT('Ctrl Pts',(0.458090774579739,-0.0559238546714361,
0.32273079639211));
#10256=CARTESIAN_POINT('Ctrl Pts',(0.359454280516197,-0.0503913533949749,
0.437723219000871));
#10257=CARTESIAN_POINT('Ctrl Pts',(0.159982027216266,-0.0401510462235837,
0.555571920770604));
#10258=CARTESIAN_POINT('Ctrl Pts',(-0.144657756582305,-0.0280423528175961,
0.579648625746246));
#10259=CARTESIAN_POINT('Ctrl Pts',(-0.492877605581078,-0.0114279703349173,
0.365435433134162));
#10260=CARTESIAN_POINT('Ctrl Pts',(-0.627676086705552,0.00672662241611611,
-0.0819941369368146));
#10261=CARTESIAN_POINT('Ctrl Pts',(-0.429575578790989,0.0217374029865393,
-0.411892296658343));
#10262=CARTESIAN_POINT('Ctrl Pts',(-0.152541695249049,0.0350886859058673,
-0.56523975267364));
#10263=CARTESIAN_POINT('Ctrl Pts',(0.135336383264751,0.0468071272484516,
-0.593307263800836));
#10264=CARTESIAN_POINT('Ctrl Pts',(0.458283899799568,0.0619230940080691,
-0.402587697314557));
#10265=CARTESIAN_POINT('Ctrl Pts',(0.609307758332133,0.077097462503894,
-0.0592237153848371));
#10266=CARTESIAN_POINT('Ctrl Pts',(0.53091310472218,0.0923272352205907,
0.30951522266531));
#10267=CARTESIAN_POINT('Ctrl Pts',(0.250724840721133,0.107614236320416,
0.56358297032994));
#10268=CARTESIAN_POINT('Ctrl Pts',(-0.126564120826802,0.122958232514227,
0.606014156402225));
#10269=CARTESIAN_POINT('Ctrl Pts',(-0.458600282429894,0.138360004467555,
0.419510886459279));
#10270=CARTESIAN_POINT('Ctrl Pts',(-0.61983176300993,0.153819591463941,
0.0719351225364332));
#10271=CARTESIAN_POINT('Ctrl Pts',(-0.554725504055214,0.167613443003585,
-0.26206181260559));
#10272=CARTESIAN_POINT('Ctrl Pts',(-0.310462228378986,0.18317983125893,
-0.547935611146063));
#10273=CARTESIAN_POINT('Ctrl Pts',(0.0780396026352433,0.198804639175307,
-0.641883892892221));
#10274=CARTESIAN_POINT('Ctrl Pts',(0.402026461102164,0.213627244123688,
-0.466519201503654));
#10275=CARTESIAN_POINT('Ctrl Pts',(0.544500361878148,0.224119082495714,
-0.261427818401927));
#10276=CARTESIAN_POINT('Ctrl Pts',(0.631628180764258,0.236382465082763,
0.0179423588092262));
#10277=CARTESIAN_POINT('Ctrl Pts',(0.516068994702346,0.253084696239743,
0.43193949622819));
#10278=CARTESIAN_POINT('Ctrl Pts',(0.0830210067449421,0.271930051773854,
0.646718419920737));
#10279=CARTESIAN_POINT('Ctrl Pts',(-0.312319178997566,0.288487979610228,
0.553307648248391));
#10280=CARTESIAN_POINT('Ctrl Pts',(-0.558279343154951,0.302727304137082,
0.307199029471688));
#10281=CARTESIAN_POINT('Ctrl Pts',(-0.653150400467482,0.319394308864648,
-0.0905802609109041));
#10282=CARTESIAN_POINT('Ctrl Pts',(-0.435122300634288,0.338520769864014,
-0.530070043401227));
#10283=CARTESIAN_POINT('Ctrl Pts',(0.100253391623782,0.360142020853588,
-0.681852822886023));
#10284=CARTESIAN_POINT('Ctrl Pts',(0.574125670286231,0.381867358768597,
-0.386613915232585));
#10285=CARTESIAN_POINT('Ctrl Pts',(0.675859963797566,0.403696019921949,
0.164969837630149));
#10286=CARTESIAN_POINT('Ctrl Pts',(0.333933833613938,0.425627009534933,
0.614092428525758));
#10287=CARTESIAN_POINT('Ctrl Pts',(-0.166855205845708,0.445212279958248,
0.65692348919662));
#10288=CARTESIAN_POINT('Ctrl Pts',(-0.512558158344907,0.462413615711228,
0.415370766303966));
#10289=CARTESIAN_POINT('Ctrl Pts',(-0.656905926926602,0.477202142388953,
0.0837178575488728));
#10290=CARTESIAN_POINT('Ctrl Pts',(-0.603934505805005,0.492035035282177,
-0.275965254620774));
#10291=CARTESIAN_POINT('Ctrl Pts',(-0.369111319436882,0.506911682404455,
-0.554385455958002));
#10292=CARTESIAN_POINT('Ctrl Pts',(-0.0215858718780792,0.521830986548816,
-0.667388550146379));
#10293=CARTESIAN_POINT('Ctrl Pts',(0.304496254884779,0.535546504631584,
-0.587631913783192));
#10294=CARTESIAN_POINT('Ctrl Pts',(0.529545529977474,0.548045825828215,
-0.387548801059109));
#10295=CARTESIAN_POINT('Ctrl Pts',(0.623430443923589,0.557440707689041,
-0.181835303568542));
#10296=CARTESIAN_POINT('Ctrl Pts',(0.654525025820574,0.568730207876573,
0.0836616613355354));
#10297=CARTESIAN_POINT('Ctrl Pts',(0.546500532924433,0.583818709910893,
0.44112976816762));
#10298=CARTESIAN_POINT('Ctrl Pts',(0.0884276227330822,0.604628824848464,
0.717869648196326));
#10299=CARTESIAN_POINT('Ctrl Pts',(-0.303138377589476,0.620555783445757,
0.601189590057862));
#10300=CARTESIAN_POINT('Ctrl Pts',(-0.459533951528957,0.629587879697291,
0.456235628332994));
#10301=CARTESIAN_POINT('Ctrl Pts',(-0.50533803825867,0.632441864943015,
0.406825610307984));
#10302=CARTESIAN_POINT('Ctrl Pts',(-0.574730547818871,0.637413806305203,
0.311344471281228));
#10303=CARTESIAN_POINT('Ctrl Pts',(-0.668366929241738,0.647578784537745,
0.0911858923259072));
#10304=CARTESIAN_POINT('Ctrl Pts',(-0.646014473739158,0.65869166785039,
-0.191884936486334));
#10305=CARTESIAN_POINT('Ctrl Pts',(-0.507750145831133,0.670756048992164,
-0.426018471870812));
#10306=CARTESIAN_POINT('Ctrl Pts',(-0.373964063037016,0.677176230628601,
-0.540642005287599));
#10307=CARTESIAN_POINT('Ctrl Pts',(-0.254981157617524,0.683225428963242,
-0.603522442720417));
#10308=CARTESIAN_POINT('Ctrl Pts',(-0.131378135817476,0.690256652979596,
-0.644880665656916));
#10309=CARTESIAN_POINT('Ctrl Pts',(0.0329691754781826,0.696925078957068,
-0.658603602643401));
#10310=CARTESIAN_POINT('Ctrl Pts',(0.286311574187696,0.695426723316108,
-0.654719844645462));
#10311=CARTESIAN_POINT('Ctrl Pts',(0.544469594489569,0.693381861459456,
-0.651898559429127));
#10312=CARTESIAN_POINT('Ctrl Pts',(0.779152740415451,0.69469615002134,-0.653791516275892));
#10313=CARTESIAN_POINT('Ctrl Pts',(1.1039892584626,0.694787852059779,-0.653948652768477));
#10314=CARTESIAN_POINT('Ctrl Pts',(1.51465812889679,0.694162579938424,-0.653012801319326));
#10315=CARTESIAN_POINT('Ctrl Pts',(1.83619183360445,0.694715125341329,-0.653830098307572));
#10316=CARTESIAN_POINT('Ctrl Pts',(2.00001383877787,0.69454111576742,-0.653575174848417));
#10317=CARTESIAN_POINT('Ctrl Pts',(0.584637750521914,-0.08002395673696,
-2.00006109519124));
#10318=CARTESIAN_POINT('Ctrl Pts',(0.584892738797937,-0.0801980105577937,
-1.8361974307128));
#10319=CARTESIAN_POINT('Ctrl Pts',(0.584070397282088,-0.0796469480362867,
-1.51453692100759));
#10320=CARTESIAN_POINT('Ctrl Pts',(0.585018211080981,-0.0802707046782126,
-1.1041699139982));
#10321=CARTESIAN_POINT('Ctrl Pts',(0.584844996796074,-0.0801826160882838,
-0.778992437761296));
#10322=CARTESIAN_POINT('Ctrl Pts',(0.582985364027564,-0.0788618850869893,
-0.544357823369232));
#10323=CARTESIAN_POINT('Ctrl Pts',(0.585729490711569,-0.0809239026814745,
-0.287182445226095));
#10324=CARTESIAN_POINT('Ctrl Pts',(0.589793240758398,-0.0823871514823907,
-0.0312569796179479));
#10325=CARTESIAN_POINT('Ctrl Pts',(0.575734031344313,-0.0758293347541534,
0.127340192047422));
#10326=CARTESIAN_POINT('Ctrl Pts',(0.53929719150208,-0.0696886811244117,
0.235037197670799));
#10327=CARTESIAN_POINT('Ctrl Pts',(0.483661895232482,-0.0643117779926539,
0.34091138833042));
#10328=CARTESIAN_POINT('Ctrl Pts',(0.379664997426553,-0.0584729700266611,
0.462212370815084));
#10329=CARTESIAN_POINT('Ctrl Pts',(0.168542708401427,-0.047636339134619,
0.587046009527204));
#10330=CARTESIAN_POINT('Ctrl Pts',(-0.152794966025498,-0.0348665665151376,
0.612175506111687));
#10331=CARTESIAN_POINT('Ctrl Pts',(-0.520842009334159,-0.0173073404504013,
0.386082361511922));
#10332=CARTESIAN_POINT('Ctrl Pts',(-0.663102892972978,0.00186395157458001,
-0.0866757237069638));
#10333=CARTESIAN_POINT('Ctrl Pts',(-0.453880008015841,0.0177235441027429,
-0.43515135255674));
#10334=CARTESIAN_POINT('Ctrl Pts',(-0.16119947896275,0.0318277200001107,
-0.597156692749208));
#10335=CARTESIAN_POINT('Ctrl Pts',(0.142901948310622,0.0442065744211116,
-0.626805484406487));
#10336=CARTESIAN_POINT('Ctrl Pts',(0.484028873946432,0.0601725007801429,
-0.425346166029852));
#10337=CARTESIAN_POINT('Ctrl Pts',(0.64352739507206,0.076198816494571,-0.0626916547305078));
#10338=CARTESIAN_POINT('Ctrl Pts',(0.560732644738571,0.0922807699482088,
0.326694597075312));
#10339=CARTESIAN_POINT('Ctrl Pts',(0.264900550785045,0.10842022799673,0.594929934911429));
#10340=CARTESIAN_POINT('Ctrl Pts',(-0.133349595055407,0.124616065358542,
0.639702884880681));
#10341=CARTESIAN_POINT('Ctrl Pts',(-0.483729766009194,0.140868429202419,
0.44287706510078));
#10342=CARTESIAN_POINT('Ctrl Pts',(-0.653802167228336,0.157176940491362,
0.0761921198620269));
#10343=CARTESIAN_POINT('Ctrl Pts',(-0.585125253714795,0.1717230801425,-0.276029079282174));
#10344=CARTESIAN_POINT('Ctrl Pts',(-0.327594459642905,0.188133786310116,
-0.577413377015519));
#10345=CARTESIAN_POINT('Ctrl Pts',(0.0818436386059794,0.204599843588814,
-0.676376077840266));
#10346=CARTESIAN_POINT('Ctrl Pts',(0.42307468801898,0.220211419499024,-0.491639799509712));
#10347=CARTESIAN_POINT('Ctrl Pts',(0.573088642458679,0.231258603176657,
-0.275687846185668));
#10348=CARTESIAN_POINT('Ctrl Pts',(0.664802204520714,0.244168010899022,
0.0184100054477792));
#10349=CARTESIAN_POINT('Ctrl Pts',(0.543155274881692,0.261739774606017,
0.453979428564444));
#10350=CARTESIAN_POINT('Ctrl Pts',(0.0878072781540096,0.281553832833368,
0.679729956787184));
#10351=CARTESIAN_POINT('Ctrl Pts',(-0.327583247797146,0.298951444403642,
0.581549148575783));
#10352=CARTESIAN_POINT('Ctrl Pts',(-0.585861055188208,0.313904711917007,
0.32307448664383));
#10353=CARTESIAN_POINT('Ctrl Pts',(-0.685400477254159,0.331397420979625,
-0.0944339892530362));
#10354=CARTESIAN_POINT('Ctrl Pts',(-0.456648649194199,0.351455627659057,
-0.555317863446294));
#10355=CARTESIAN_POINT('Ctrl Pts',(0.104355064344254,0.374109670982164,
-0.714240744447354));
#10356=CARTESIAN_POINT('Ctrl Pts',(0.600325552444107,0.396850329478333,
-0.40508685912858));
#10357=CARTESIAN_POINT('Ctrl Pts',(0.706584395423094,0.419675484364605,
0.171729518407216));
#10358=CARTESIAN_POINT('Ctrl Pts',(0.34930514669001,0.44258333888256,0.640786410100714));
#10359=CARTESIAN_POINT('Ctrl Pts',(-0.17322023746871,0.463017272571361,
0.685360699154325));
#10360=CARTESIAN_POINT('Ctrl Pts',(-0.533554981839275,0.480948121262819,
0.433520010328514));
#10361=CARTESIAN_POINT('Ctrl Pts',(-0.683875307228172,0.496351419981493,
0.0880553591433872));
#10362=CARTESIAN_POINT('Ctrl Pts',(-0.628700661609138,0.511787915912003,
-0.28627172728474));
#10363=CARTESIAN_POINT('Ctrl Pts',(-0.384483316527052,0.527257112128013,
-0.575768939686068));
#10364=CARTESIAN_POINT('Ctrl Pts',(-0.0233796950368831,0.542758397070066,
-0.693135592308099));
#10365=CARTESIAN_POINT('Ctrl Pts',(0.315129613443997,0.556996626383038,
-0.610300901439449));
#10366=CARTESIAN_POINT('Ctrl Pts',(0.548563681096053,0.569962296360195,
-0.402727787084418));
#10367=CARTESIAN_POINT('Ctrl Pts',(0.645875656884303,0.579701111353387,
-0.189469234165643));
#10368=CARTESIAN_POINT('Ctrl Pts',(0.678087402227607,0.591399053727189,
0.0856332935540037));
#10369=CARTESIAN_POINT('Ctrl Pts',(0.566180342756128,0.607021306882514,
0.455764435882692));
#10370=CARTESIAN_POINT('Ctrl Pts',(0.0923367089252467,0.628543104862909,
0.741820632313748));
#10371=CARTESIAN_POINT('Ctrl Pts',(-0.311985282045994,0.644989463074714,
0.621215254019459));
#10372=CARTESIAN_POINT('Ctrl Pts',(-0.473404249561221,0.654311438758149,
0.47160992481743));
#10373=CARTESIAN_POINT('Ctrl Pts',(-0.520670030114206,0.65725685157747,
0.420614920065451));
#10374=CARTESIAN_POINT('Ctrl Pts',(-0.592248587258343,0.662383411221966,
0.322168780482819));
#10375=CARTESIAN_POINT('Ctrl Pts',(-0.688734911720638,0.672871119021292,
0.0950038824064079));
#10376=CARTESIAN_POINT('Ctrl Pts',(-0.665867604510835,0.684306259795084,
-0.196319960324102));
#10377=CARTESIAN_POINT('Ctrl Pts',(-0.523264547581101,0.696742034629231,
-0.43769269867827));
#10378=CARTESIAN_POINT('Ctrl Pts',(-0.385571678876014,0.703352498122265,
-0.555622128823214));
#10379=CARTESIAN_POINT('Ctrl Pts',(-0.263639834025884,0.709548173405927,
-0.620061658738199));
#10380=CARTESIAN_POINT('Ctrl Pts',(-0.13596345065982,0.716817624310851,
-0.662808505090214));
#10381=CARTESIAN_POINT('Ctrl Pts',(0.0328701126263124,0.723623474439416,
-0.67673682834849));
#10382=CARTESIAN_POINT('Ctrl Pts',(0.286974825485283,0.722084330497799,
-0.672795432729989));
#10383=CARTESIAN_POINT('Ctrl Pts',(0.544470548836667,0.720058117306266,
-0.669996370718004));
#10384=CARTESIAN_POINT('Ctrl Pts',(0.778866262009698,0.721364810413718,
-0.671878222247616));
#10385=CARTESIAN_POINT('Ctrl Pts',(1.10424366248717,0.721460534244764,-0.672039567606643));
#10386=CARTESIAN_POINT('Ctrl Pts',(1.51446664209188,0.72083249825408,-0.671098379809243));
#10387=CARTESIAN_POINT('Ctrl Pts',(1.83619853648755,0.721386379956638,-0.671916335232525));
#10388=CARTESIAN_POINT('Ctrl Pts',(2.00007031245355,0.72121231751685,-0.671661334325028));
#10389=CARTESIAN_POINT('Ctrl Pts',(0.600124355483138,-0.0799998580128369,
-2.00008516830249));
#10390=CARTESIAN_POINT('Ctrl Pts',(0.600379376695529,-0.0801739343158842,
-1.83620033785433));
#10391=CARTESIAN_POINT('Ctrl Pts',(0.599557188536607,-0.0796220546015198,
-1.51445131895255));
#10392=CARTESIAN_POINT('Ctrl Pts',(0.60050657815397,-0.0802473516234908,
-1.10427966986787));
#10393=CARTESIAN_POINT('Ctrl Pts',(0.600332768539301,-0.0801568850586992,
-0.778861249100346));
#10394=CARTESIAN_POINT('Ctrl Pts',(0.598475600091931,-0.078840606257744,
-0.544366061842844));
#10395=CARTESIAN_POINT('Ctrl Pts',(0.601215825651616,-0.0808915608655967,
-0.287431516632137));
#10396=CARTESIAN_POINT('Ctrl Pts',(0.605291661148957,-0.0823787912019986,
-0.0313608552946517));
#10397=CARTESIAN_POINT('Ctrl Pts',(0.59116069745846,-0.0757414785640243,
0.130026789470337));
#10398=CARTESIAN_POINT('Ctrl Pts',(0.553569673303418,-0.0693986540389958,
0.241244525168603));
#10399=CARTESIAN_POINT('Ctrl Pts',(0.49648068595625,-0.0638861429178919,
0.349817593838996));
#10400=CARTESIAN_POINT('Ctrl Pts',(0.389834766749766,-0.0578962864213881,
0.474234392676377));
#10401=CARTESIAN_POINT('Ctrl Pts',(0.172953767301598,-0.0467647821330201,
0.602517389648945));
#10402=CARTESIAN_POINT('Ctrl Pts',(-0.156611161701388,-0.033669257315275,
0.62816084010969));
#10403=CARTESIAN_POINT('Ctrl Pts',(-0.534324881784356,-0.0156487609275952,
0.396251684871875));
#10404=CARTESIAN_POINT('Ctrl Pts',(-0.680173923436771,0.00401467962268951,
-0.0887673006211078));
#10405=CARTESIAN_POINT('Ctrl Pts',(-0.465603920420951,0.020280840108104,
-0.446125545894049));
#10406=CARTESIAN_POINT('Ctrl Pts',(-0.16548447812985,0.0347430378954353,
-0.612246576434715));
#10407=CARTESIAN_POINT('Ctrl Pts',(0.146296739212227,0.0474345780356556,
-0.642633153997123));
#10408=CARTESIAN_POINT('Ctrl Pts',(0.495951952987202,0.063799790307997,
-0.436120013454043));
#10409=CARTESIAN_POINT('Ctrl Pts',(0.659386574747031,0.0802231528742134,
-0.0644747476625062));
#10410=CARTESIAN_POINT('Ctrl Pts',(0.574545975795925,0.0966991624308195,
0.334451049923668));
#10411=CARTESIAN_POINT('Ctrl Pts',(0.271532980288635,0.11322968614674,0.60917227723542));
#10412=CARTESIAN_POINT('Ctrl Pts',(-0.136251703472976,0.12981319447486,
0.654997709328214));
#10413=CARTESIAN_POINT('Ctrl Pts',(-0.494901469661726,0.146449568036652,
0.45350333530914));
#10414=CARTESIAN_POINT('Ctrl Pts',(-0.668917235906318,0.163138202692549,
0.0782626975824873));
#10415=CARTESIAN_POINT('Ctrl Pts',(-0.598645464166764,0.178018515644393,
-0.282045078558144));
#10416=CARTESIAN_POINT('Ctrl Pts',(-0.335262469427464,0.194801446585974,
-0.590258155385672));
#10417=CARTESIAN_POINT('Ctrl Pts',(0.0833245701146875,0.211635076942448,
-0.691392401965039));
#10418=CARTESIAN_POINT('Ctrl Pts',(0.432010324368538,0.227588445577569,
-0.502588887028728));
#10419=CARTESIAN_POINT('Ctrl Pts',(0.585260109788594,0.238874210076111,
-0.281973448384831));
#10420=CARTESIAN_POINT('Ctrl Pts',(0.678932070081789,0.25205984880311,0.018422105283869));
#10421=CARTESIAN_POINT('Ctrl Pts',(0.55467369883675,0.270001497383997,0.463140844788188));
#10422=CARTESIAN_POINT('Ctrl Pts',(0.0899761556469263,0.290221466632431,
0.693463094883412));
#10423=CARTESIAN_POINT('Ctrl Pts',(-0.33371627867329,0.307967186991324,
0.593293078602062));
#10424=CARTESIAN_POINT('Ctrl Pts',(-0.59704764533906,0.323213852266529,
0.329736222807235));
#10425=CARTESIAN_POINT('Ctrl Pts',(-0.698474654722095,0.341042833941317,
-0.0958055766422671));
#10426=CARTESIAN_POINT('Ctrl Pts',(-0.465383647491834,0.361476669823075,
-0.565288791036093));
#10427=CARTESIAN_POINT('Ctrl Pts',(0.105790956320368,0.384540697804113,
-0.727009690342144));
#10428=CARTESIAN_POINT('Ctrl Pts',(0.610371558079431,0.407678360937913,
-0.412394382377907));
#10429=CARTESIAN_POINT('Ctrl Pts',(0.718333583382585,0.43088704560672,0.174123208014002));
#10430=CARTESIAN_POINT('Ctrl Pts',(0.355226639142397,0.454164351268278,
0.650688896190773));
#10431=CARTESIAN_POINT('Ctrl Pts',(-0.17537106718635,0.474914221668976,
0.695875511358292));
#10432=CARTESIAN_POINT('Ctrl Pts',(-0.54103585275066,0.493111378816631,
0.440272937100537));
#10433=CARTESIAN_POINT('Ctrl Pts',(-0.6934950282823,0.508736295299708,0.0898302457491503));
#10434=CARTESIAN_POINT('Ctrl Pts',(-0.637526970610404,0.524387740772898,
-0.289700706598419));
#10435=CARTESIAN_POINT('Ctrl Pts',(-0.390008311550144,0.540064979323309,
-0.583068679337088));
#10436=CARTESIAN_POINT('Ctrl Pts',(-0.024226148296103,0.555766910199861,
-0.701929930807063));
#10437=CARTESIAN_POINT('Ctrl Pts',(0.318491600824293,0.570182538995617,
-0.618039769051569));
#10438=CARTESIAN_POINT('Ctrl Pts',(0.554723176441453,0.583304202833105,
-0.40796362014035));
#10439=CARTESIAN_POINT('Ctrl Pts',(0.653160192073423,0.593156620195102,
-0.192217361281352));
#10440=CARTESIAN_POINT('Ctrl Pts',(0.685736178259883,0.60498732605382,0.0860074066354565));
#10441=CARTESIAN_POINT('Ctrl Pts',(0.572562677668091,0.620781559492554,
0.4602016432688));
#10442=CARTESIAN_POINT('Ctrl Pts',(0.0937765103860463,0.642526123974182,
0.7491364099364));
#10443=CARTESIAN_POINT('Ctrl Pts',(-0.314388630844237,0.659130029858254,
0.627315372568153));
#10444=CARTESIAN_POINT('Ctrl Pts',(-0.477285810697724,0.668537384089933,
0.47634220294986));
#10445=CARTESIAN_POINT('Ctrl Pts',(-0.524979531484106,0.671509580653182,
0.42488265802704));
#10446=CARTESIAN_POINT('Ctrl Pts',(-0.597194271883867,0.676681179673865,
0.325573954028726));
#10447=CARTESIAN_POINT('Ctrl Pts',(-0.694496329532521,0.687262154305694,
0.0963821879712936));
#10448=CARTESIAN_POINT('Ctrl Pts',(-0.671478629812927,0.698788430555515,
-0.197261795472992));
#10449=CARTESIAN_POINT('Ctrl Pts',(-0.527677507863671,0.71132631016803,
-0.440626908636377));
#10450=CARTESIAN_POINT('Ctrl Pts',(-0.388905141275015,0.717990004861966,
-0.559470705037612));
#10451=CARTESIAN_POINT('Ctrl Pts',(-0.266282257094333,0.724219498671225,
-0.624266154108112));
#10452=CARTESIAN_POINT('Ctrl Pts',(-0.13757925918983,0.731550254164043,
-0.667380131292113));
#10453=CARTESIAN_POINT('Ctrl Pts',(0.0327675186379925,0.738404779593333,
-0.681400099587548));
#10454=CARTESIAN_POINT('Ctrl Pts',(0.28724639971344,0.736851511264604,-0.677433025330373));
#10455=CARTESIAN_POINT('Ctrl Pts',(0.544462158077268,0.734831948662016,
-0.674646491228074));
#10456=CARTESIAN_POINT('Ctrl Pts',(0.778748964711316,0.736136065865045,
-0.676524055782765));
#10457=CARTESIAN_POINT('Ctrl Pts',(1.10434282010243,0.736233268880018,-0.676688327154564));
#10458=CARTESIAN_POINT('Ctrl Pts',(1.51438929680924,0.735604358561319,-0.675746079653723));
#10459=CARTESIAN_POINT('Ctrl Pts',(1.83620130898864,0.736158775205925,-0.676565295388705));
#10460=CARTESIAN_POINT('Ctrl Pts',(2.00009323767342,0.735984691360185,-0.676310263121558));
#10461=CARTESIAN_POINT('Origin',(0.6,0.,-2.));
#10462=CARTESIAN_POINT('Origin',(1.99999999999998,0.759999999999999,-0.60000000000007));
#10463=CARTESIAN_POINT('Origin',(1.99999999999998,0.759999999999999,-0.60000000000007));
#10464=CARTESIAN_POINT('Origin',(0.6,0.,-2.));
#11218=UNCERTAINTY_MEASURE_WITH_UNIT(LENGTH_MEASURE(0.001),#11259,
'DISTANCE_ACCURACY_VALUE',
'Maximum model space distance between geometric entities at asserted c
onnectivities');
#11228=UNCERTAINTY_MEASURE_WITH_UNIT(LENGTH_MEASURE(0.001),#11259,
'DISTANCE_ACCURACY_VALUE',
'Maximum model space distance between geometric entities at asserted c
onnectivities');
#11248=(
GEOMETRIC_REPRESENTATION_CONTEXT(3)
GLOBAL_UNCERTAINTY_ASSIGNED_CONTEXT((#11218))
GLOBAL_UNIT_ASSIGNED_CONTEXT((#11259,#11261,#11262))
REPRESENTATION_CONTEXT('','3D')
);
#11258=(
GEOMETRIC_REPRESENTATION_CONTEXT(3)
GLOBAL_UNCERTAINTY_ASSIGNED_CONTEXT((#11228))
GLOBAL_UNIT_ASSIGNED_CONTEXT((#11259,#11261,#11262))
REPRESENTATION_CONTEXT('','3D')
);
#11259=(
LENGTH_UNIT()
NAMED_UNIT(*)
SI_UNIT(.CENTI.,.METRE.)
);
#11261=(
NAMED_UNIT(*)
PLANE_ANGLE_UNIT()
SI_UNIT($,.RADIAN.)
);
#11262=(
NAMED_UNIT(*)
SI_UNIT($,.STERADIAN.)
SOLID_ANGLE_UNIT()
);
#11282=SHAPE_DEFINITION_REPRESENTATION(#11316,#11378);
#11316=PRODUCT_DEFINITION_SHAPE('',$,#11408);
#11378=SHAPE_REPRESENTATION('',(#5862),#11248);
#11388=PRODUCT_DEFINITION_CONTEXT('part definition',#11477,'design');
#11408=PRODUCT_DEFINITION(
'Torsion Spring - 1.6 mm Wire, 12 mm Coil, 4.75 Turns',
'Torsion Spring - 1.6 mm Wire, 12 mm Coil, 4.75 Turns',#11437,#11388);
#11437=PRODUCT_DEFINITION_FORMATION('',$,#11498);
#11477=APPLICATION_CONTEXT(
'Core Data for Automotive Mechanical Design Process');
#11478=PRODUCT_CONTEXT('part definition',#11477,'mechanical');
#11498=PRODUCT('Torsion Spring - 1.6 mm Wire, 12 mm Coil, 4.75 Turns',
'Torsion Spring - 1.6 mm Wire, 12 mm Coil, 4.75 Turns',
'Torsion Spring - 1.6 mm Wire, 12 mm Coil, 4.75 Turns',(#11478));
#11578=COLOUR_RGB('Grey',0.48,0.52,0.57);
#11579=FILL_AREA_STYLE_COLOUR('',#11578);
#11580=FILL_AREA_STYLE('',(#11579));
#11581=SURFACE_STYLE_FILL_AREA(#11580);
#11582=SURFACE_SIDE_STYLE('',(#11581));
#11583=SURFACE_STYLE_USAGE(.BOTH.,#11582);
#11584=PRESENTATION_STYLE_ASSIGNMENT((#11583));
ENDSEC;
END-ISO-10303-21;
